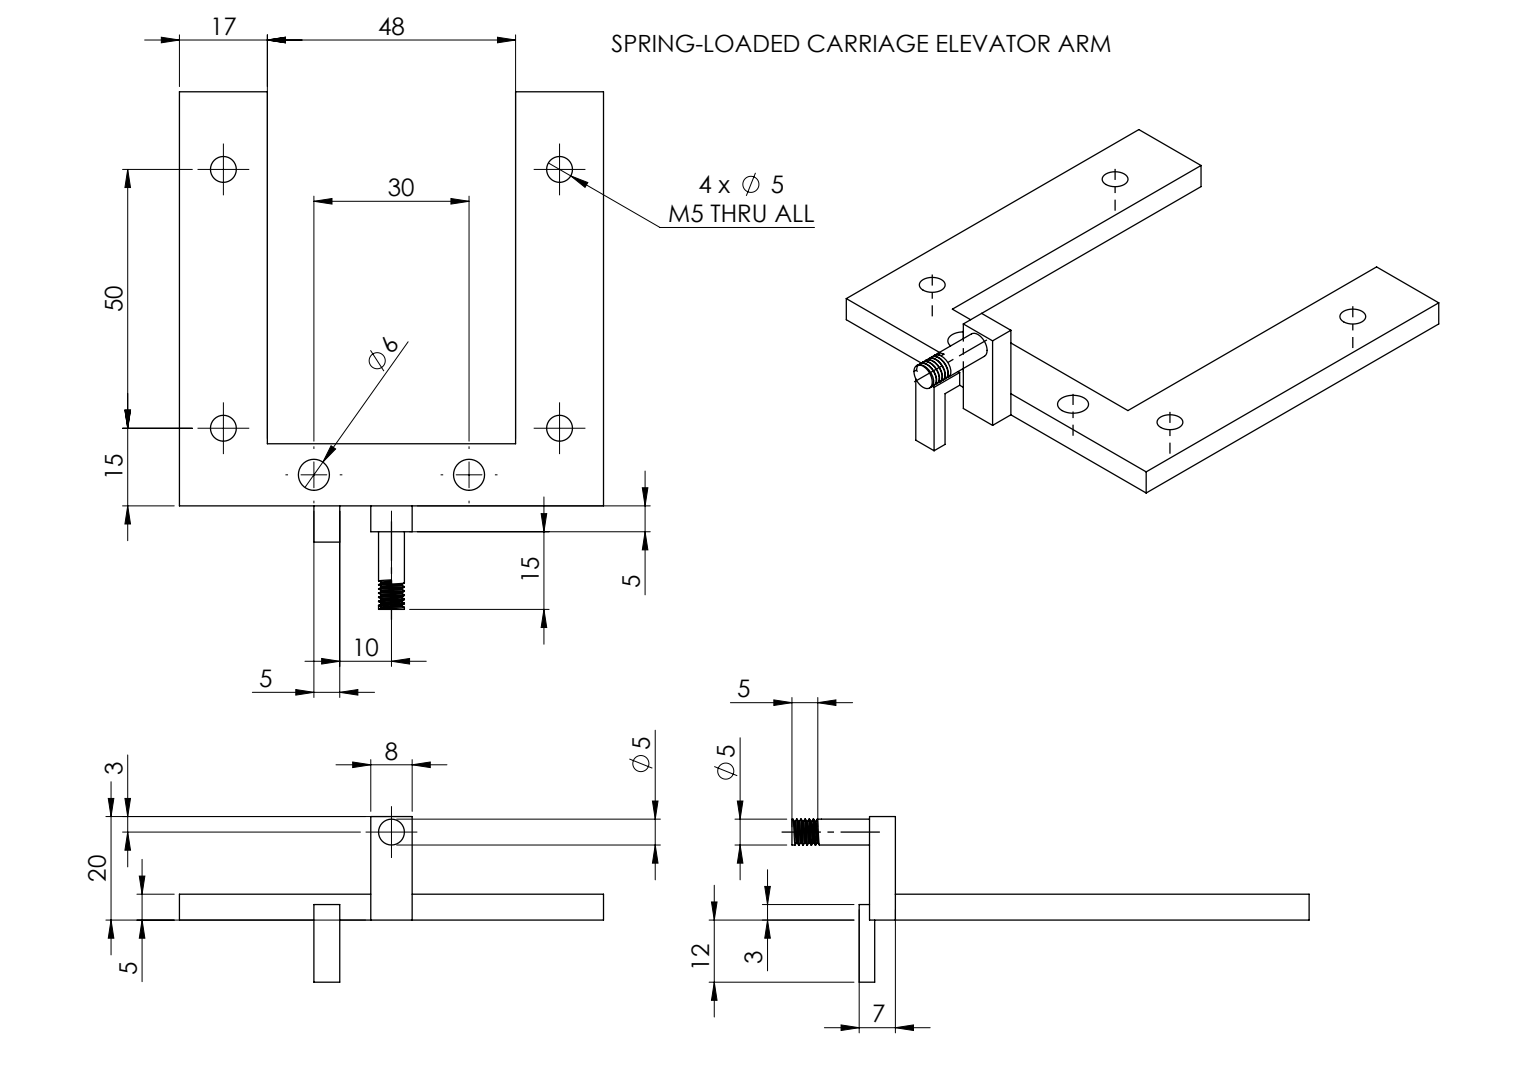
ISO-10303-21;
HEADER;
FILE_DESCRIPTION (('STEP AP214'),
    '1' );
FILE_NAME ('Spring-Loaded Carriage Elevator Arm.step',
    '2026-10-08T14:41:38',
    ( '' ),
    ( '' ),
    'SwSTEP 2.0',
    'SolidWorks 2026',
    '' );
FILE_SCHEMA (( 'AUTOMOTIVE_DESIGN' ));
ENDSEC;

DATA;
#4=DIRECTION ( 'NONE',  ( -0.000000000000000000, 1.000000000000000000, -0.000000000000000000 ) ) ;
#23=DIRECTION ( 'NONE',  ( -0.000000000000000000, -0.000000000000000000, -1.000000000000000000 ) ) ;
#28=CARTESIAN_POINT ( 'NONE',  ( -2.066987300000001415, 63.14382582708705627, 44.80000000109247082 ) ) ;
#31=ORIENTED_EDGE ( 'NONE', *, *, #8748, .T. ) ;
#34=ORIENTED_EDGE ( 'NONE', *, *, #9742, .F. ) ;
#41=CARTESIAN_POINT ( 'NONE',  ( 1.461580736456473684, 65.46158073645646880, 45.45000000109246940 ) ) ;
#50=AXIS2_PLACEMENT_3D ( 'NONE', #5480, #14305, #2436 ) ;
#54=CARTESIAN_POINT ( 'NONE',  ( 1.767766952966369987, 65.76776695296638309, 49.00000000218494023 ) ) ;
#57=EDGE_CURVE ( 'NONE', #1624, #17649, #87, .T. ) ;
#58=CARTESIAN_POINT ( 'NONE',  ( 2.066987300000002303, 63.14382582708705627, 45.30000000109247082 ) ) ;
#68=FACE_OUTER_BOUND ( 'NONE', #2154, .T. ) ;
#73=ORIENTED_EDGE ( 'NONE', *, *, #1505, .T. ) ;
#80=FACE_OUTER_BOUND ( 'NONE', #9007, .T. ) ;
#84=ORIENTED_EDGE ( 'NONE', *, *, #1267, .T. ) ;
#87=LINE ( 'NONE', #2922, #12898 ) ;
#104=CARTESIAN_POINT ( 'NONE',  ( -1.767766952966370209, 65.76776695296638309, 45.09999999999999432 ) ) ;
#108=CARTESIAN_POINT ( 'NONE',  ( 1.035533905932738197, 66.50000000000000000, 47.45000000218494307 ) ) ;
#117=( BOUNDED_SURFACE ( )  B_SPLINE_SURFACE ( 1, 2, ( 
 ( #9163, #1629, #4271, #7495, #8867, #13566, #54, #147, #16622, #6038, #10621, #5837, #11801, #11995, #17795, #6132, #7697, #11700, #4368, #8766, #10328, #18092, #13663, #17993, #16519, #4567, #7300, #3082, #9063, #3189, #15146, #1716, #14852, #17693, #14756, #16325, #2892, #12485, #3479, #12194, #442, #7902, #14057, #8092, #12393, #13866, #14158, #7997, #9347, #18390, #537, #2108, #16718, #6621, #631, #6520, #347, #6427, #4959, #12590, #4862, #4774, #15339, #1815, #3572, #3380, #18195, #18582, #10724, #1916, #2196, #10915, #5055, #16914, #7795, #9453, #10818, #16816, #5148, #11110, #11015, #17106, #3286, #13963, #15243, #15441, #9257, #13766, #15626, #18487, #2006, #6333, #12299, #15537, #18294, #17014, #3670, #9545, #9641, #8190, #6229 ),
 ( #18952, #2384, #1012, #18680, #11198, #18866, #15731, #11580, #14338, #911, #11481, #3953, #5519, #3859, #728, #2668, #5428, #9821, #6987, #17378, #6707, #6893, #8369, #8555, #2573, #12865, #11386, #8648, #2474, #15818, #9915, #14438, #16015, #17201, #1102, #14530, #12953, #14247, #15910, #8462, #7083, #18763, #5245, #17469, #2291, #4045, #17293, #12678, #13046, #3766, #10011, #16101, #19045, #5618, #17578, #8277, #4155, #5336, #11297, #10105, #9735, #818, #6803, #12767, #2961, #4248, #7378, #13151, #17669, #4646, #7471, #2867, #14730, #10206, #4543, #16197, #1401, #10502, #1308, #8739, #4344, #15028, #11876, #7281, #16500, #9040, #13444, #16295, #14933, #19149, #5720, #13349, #2764, #6109, #13247, #28, #19343, #10403, #19244, #1504, #12075 ) ),
 .UNSPECIFIED., .F., .F., .F. ) 
 B_SPLINE_SURFACE_WITH_KNOTS ( ( 2, 2 ),
 ( 3, 2, 2, 2, 2, 2, 2, 2, 2, 2, 2, 2, 2, 2, 2, 2, 2, 2, 2, 2, 2, 2, 2, 2, 2, 2, 2, 2, 2, 2, 2, 2, 2, 2, 2, 2, 2, 2, 2, 2, 2, 2, 2, 2, 2, 2, 2, 2, 2, 2, 3 ),
 ( 0.000000000000000000, 1.000000000000000000 ),
 ( 0.000000000000000000, 0.01785714285714285615, 0.03571428571428571230, 0.05357142857142856845, 0.07142857142857142461, 0.08928571428571428770, 0.1071428571428571369, 0.1250000000000000000, 0.1428571428571428492, 0.1607142857142857262, 0.1785714285714285754, 0.1964285714285714246, 0.2142857142857142738, 0.2321428571428571508, 0.2500000000000000000, 0.2678571428571428492, 0.2857142857142856984, 0.3035714285714285476, 0.3214285714285714524, 0.3392857142857143016, 0.3571428571428571508, 0.3750000000000000000, 0.3928571428571428492, 0.4107142857142856984, 0.4285714285714285476, 0.4464285714285714524, 0.4642857142857143016, 0.4821428571428571508, 0.5000000000000000000, 0.5178571428571429047, 0.5357142857142856984, 0.5535714285714286031, 0.5714285714285713969, 0.5892857142857143016, 0.6071428571428570953, 0.6250000000000000000, 0.6428571428571429047, 0.6607142857142856984, 0.6785714285714286031, 0.6964285714285713969, 0.7142857142857143016, 0.7321428571428570953, 0.7500000000000000000, 0.7678571428571429047, 0.7857142857142856984, 0.8035714285714286031, 0.8214285714285713969, 0.8392857142857143016, 0.8571428571428570953, 0.8750000000000000000, 0.8928571428571429047 ),
 .UNSPECIFIED. ) 
 GEOMETRIC_REPRESENTATION_ITEM ( )  RATIONAL_B_SPLINE_SURFACE ( (
 ( 1.000000000000000000, 0.9238795325112867385, 1.000000000000000000, 0.9238795325112867385, 1.000000000000000000, 0.9238795325112867385, 1.000000000000000000, 0.9238795325112867385, 1.000000000000000000, 0.9238795325112867385, 1.000000000000000000, 0.9238795325112867385, 1.000000000000000000, 0.9238795325112867385, 1.000000000000000000, 0.9238795325112867385, 1.000000000000000000, 0.9238795325112867385, 1.000000000000000000, 0.9238795325112867385, 1.000000000000000000, 0.9238795325112867385, 1.000000000000000000, 0.9238795325112867385, 1.000000000000000000, 0.9238795325112867385, 1.000000000000000000, 0.9238795325112867385, 1.000000000000000000, 0.9238795325112867385, 1.000000000000000000, 0.9238795325112867385, 1.000000000000000000, 0.9238795325112867385, 1.000000000000000000, 0.9238795325112867385, 1.000000000000000000, 0.9238795325112867385, 1.000000000000000000, 0.9238795325112867385, 1.000000000000000000, 0.9238795325112867385, 1.000000000000000000, 0.9238795325112867385, 1.000000000000000000, 0.9238795325112867385, 1.000000000000000000, 0.9238795325112867385, 1.000000000000000000, 0.9238795325112867385, 1.000000000000000000, 0.9238795325112867385, 1.000000000000000000, 0.9238795325112867385, 1.000000000000000000, 0.9238795325112867385, 1.000000000000000000, 0.9238795325112867385, 1.000000000000000000, 0.9238795325112867385, 1.000000000000000000, 0.9238795325112867385, 1.000000000000000000, 0.9238795325112867385, 1.000000000000000000, 0.9238795325112867385, 1.000000000000000000, 0.9238795325112867385, 1.000000000000000000, 0.9238795325112867385, 1.000000000000000000, 0.9238795325112867385, 1.000000000000000000, 0.9238795325112867385, 1.000000000000000000, 0.9238795325112867385, 1.000000000000000000, 0.9238795325112867385, 1.000000000000000000, 0.9238795325112867385, 1.000000000000000000, 0.9238795325112867385, 1.000000000000000000, 0.9238795325112867385, 1.000000000000000000, 0.9238795325112867385, 1.000000000000000000, 0.9238795325112867385, 1.000000000000000000, 0.9238795325112867385, 1.000000000000000000, 0.9238795325112867385, 1.000000000000000000, 0.9238795325112867385, 1.000000000000000000, 0.9238795325112867385, 1.000000000000000000, 0.9238795325112867385, 1.000000000000000000, 0.9238795325112867385, 1.000000000000000000),
 ( 1.000000000000000000, 0.9238795325112867385, 1.000000000000000000, 0.9238795325112867385, 1.000000000000000000, 0.9238795325112867385, 1.000000000000000000, 0.9238795325112867385, 1.000000000000000000, 0.9238795325112867385, 1.000000000000000000, 0.9238795325112867385, 1.000000000000000000, 0.9238795325112867385, 1.000000000000000000, 0.9238795325112867385, 1.000000000000000000, 0.9238795325112867385, 1.000000000000000000, 0.9238795325112867385, 1.000000000000000000, 0.9238795325112867385, 1.000000000000000000, 0.9238795325112867385, 1.000000000000000000, 0.9238795325112867385, 1.000000000000000000, 0.9238795325112867385, 1.000000000000000000, 0.9238795325112867385, 1.000000000000000000, 0.9238795325112867385, 1.000000000000000000, 0.9238795325112867385, 1.000000000000000000, 0.9238795325112867385, 1.000000000000000000, 0.9238795325112867385, 1.000000000000000000, 0.9238795325112867385, 1.000000000000000000, 0.9238795325112867385, 1.000000000000000000, 0.9238795325112867385, 1.000000000000000000, 0.9238795325112867385, 1.000000000000000000, 0.9238795325112867385, 1.000000000000000000, 0.9238795325112867385, 1.000000000000000000, 0.9238795325112867385, 1.000000000000000000, 0.9238795325112867385, 1.000000000000000000, 0.9238795325112867385, 1.000000000000000000, 0.9238795325112867385, 1.000000000000000000, 0.9238795325112867385, 1.000000000000000000, 0.9238795325112867385, 1.000000000000000000, 0.9238795325112867385, 1.000000000000000000, 0.9238795325112867385, 1.000000000000000000, 0.9238795325112867385, 1.000000000000000000, 0.9238795325112867385, 1.000000000000000000, 0.9238795325112867385, 1.000000000000000000, 0.9238795325112867385, 1.000000000000000000, 0.9238795325112867385, 1.000000000000000000, 0.9238795325112867385, 1.000000000000000000, 0.9238795325112867385, 1.000000000000000000, 0.9238795325112867385, 1.000000000000000000, 0.9238795325112867385, 1.000000000000000000, 0.9238795325112867385, 1.000000000000000000, 0.9238795325112867385, 1.000000000000000000, 0.9238795325112867385, 1.000000000000000000, 0.9238795325112867385, 1.000000000000000000, 0.9238795325112867385, 1.000000000000000000, 0.9238795325112867385, 1.000000000000000000, 0.9238795325112867385, 1.000000000000000000, 0.9238795325112867385, 1.000000000000000000) ) ) 
 REPRESENTATION_ITEM ( '' )  SURFACE ( )  );
#121=DIRECTION ( 'NONE',  ( -0.000000000000000000, -1.000000000000000000, -0.000000000000000000 ) ) ;
#127=DIRECTION ( 'NONE',  ( -0.000000000000000000, -0.000000000000000000, -1.000000000000000000 ) ) ;
#131=DIRECTION ( 'NONE',  ( -0.000000000000000000, -0.000000000000000000, -1.000000000000000000 ) ) ;
#137=CARTESIAN_POINT ( 'NONE',  ( -2.066987300000001415, 64.85617417291294373, 48.10000000109246798 ) ) ;
#142=ORIENTED_EDGE ( 'NONE', *, *, #12510, .F. ) ;
#147=CARTESIAN_POINT ( 'NONE',  ( 2.500000000000001776, 65.03553390593273775, 48.95000000218495018 ) ) ;
#156=CARTESIAN_POINT ( 'NONE',  ( -2.066987300000001859, 64.85617417291294373, 48.90000000109247225 ) ) ;
#159=PLANE ( 'NONE',  #4117 ) ;
#165=EDGE_CURVE ( 'NONE', #16279, #13992, #8531, .T. ) ;
#186=CARTESIAN_POINT ( 'NONE',  ( 0.000000000000000000, 47.00000000000000711, -50.00000000000000000 ) ) ;
#195=ORIENTED_EDGE ( 'NONE', *, *, #2336, .T. ) ;
#203=CARTESIAN_POINT ( 'NONE',  ( 0.8561741729129471734, 61.93301270000000613, 49.00000000109246656 ) ) ;
#204=DIRECTION ( 'NONE',  ( 0.000000000000000000, 0.000000000000000000, 1.000000000000000000 ) ) ;
#208=CARTESIAN_POINT ( 'NONE',  ( -2.500000000000001776, 64.00000000000000000, 44.50000000218494733 ) ) ;
#211=LINE ( 'NONE', #15300, #5330 ) ;
#213=CARTESIAN_POINT ( 'NONE',  ( -2.500000000000001776, 64.00000000000000000, 46.79999999999999716 ) ) ;
#215=CARTESIAN_POINT ( 'NONE',  ( -10.00000000000000000, 50.00000000000000000, 30.00000000000000000 ) ) ;
#220=CARTESIAN_POINT ( 'NONE',  ( -2.500000000000019096, 65.03553390593272354, 48.35000000000000853 ) ) ;
#225=AXIS2_PLACEMENT_3D ( 'NONE', #6440, #18405, #16930 ) ;
#227=DIRECTION ( 'NONE',  ( 0.000000000000000000, 0.000000000000000000, -1.000000000000000000 ) ) ;
#232=VERTEX_POINT ( 'NONE', #15660 ) ;
#240=CARTESIAN_POINT ( 'NONE',  ( -32.50000000000000000, 52.00000000000000711, 12.50000000000000000 ) ) ;
#251=DIRECTION ( 'NONE',  ( -0.000000000000000000, -0.000000000000000000, -1.000000000000000000 ) ) ;
#253=CARTESIAN_POINT ( 'NONE',  ( 2.066987300000001859, 64.85617417291294373, 46.20000000109247651 ) ) ;
#261=ORIENTED_EDGE ( 'NONE', *, *, #4730, .T. ) ;
#272=ORIENTED_EDGE ( 'NONE', *, *, #12825, .F. ) ;
#274=DIRECTION ( 'NONE',  ( -1.000000000000000000, 0.000000000000000000, 0.000000000000000000 ) ) ;
#292=VERTEX_POINT ( 'NONE', #6652 ) ;
#295=CARTESIAN_POINT ( 'NONE',  ( 2.066987300000001415, 64.85617417291294373, 49.20000000109247651 ) ) ;
#297=VERTEX_POINT ( 'NONE', #14188 ) ;
#307=LINE ( 'NONE', #9221, #11899 ) ;
#311=DIRECTION ( 'NONE',  ( 1.000000000000000000, 0.000000000000000000, 0.000000000000000000 ) ) ;
#318=AXIS2_PLACEMENT_3D ( 'NONE', #6383, #18632, #12346 ) ;
#323=CARTESIAN_POINT ( 'NONE',  ( -10.00000000000000000, 0.000000000000000000, 33.99999999999999289 ) ) ;
#324=ORIENTED_EDGE ( 'NONE', *, *, #4947, .F. ) ;
#333=ORIENTED_EDGE ( 'NONE', *, *, #12310, .F. ) ;
#341=DIRECTION ( 'NONE',  ( -0.000000000000000000, -1.000000000000000000, 0.000000000000000000 ) ) ;
#347=CARTESIAN_POINT ( 'NONE',  ( 2.500000000000001776, 64.00000000000000000, 46.50000000218494733 ) ) ;
#354=FACE_OUTER_BOUND ( 'NONE', #14089, .T. ) ;
#355=( GEOMETRIC_REPRESENTATION_CONTEXT ( 3 ) GLOBAL_UNCERTAINTY_ASSIGNED_CONTEXT ( ( #18086 ) ) GLOBAL_UNIT_ASSIGNED_CONTEXT ( ( #12843, #5500, #19029 ) ) REPRESENTATION_CONTEXT ( 'NONE', 'WORKASPACE' ) );
#356=CARTESIAN_POINT ( 'NONE',  ( -2.066987300000001415, 63.14382582708705627, 48.20000000109247651 ) ) ;
#362=AXIS2_PLACEMENT_3D ( 'NONE', #17371, #11102, #3758 ) ;
#375=VERTEX_POINT ( 'NONE', #7113 ) ;
#387=EDGE_CURVE ( 'NONE', #7750, #14031, #2123, .T. ) ;
#395=EDGE_LOOP ( 'NONE', ( #10179, #10468 ) ) ;
#399=CARTESIAN_POINT ( 'NONE',  ( -0.8561741729129466183, 61.93301270000000613, 47.30000000109247082 ) ) ;
#400=FACE_OUTER_BOUND ( 'NONE', #585, .T. ) ;
#406=ORIENTED_EDGE ( 'NONE', *, *, #3062, .T. ) ;
#419=ORIENTED_EDGE ( 'NONE', *, *, #16592, .T. ) ;
#420=EDGE_CURVE ( 'NONE', #9430, #8882, #10133, .T. ) ;
#434=DIRECTION ( 'NONE',  ( -0.000000000000000000, 1.000000000000000000, -0.000000000000000000 ) ) ;
#439=UNCERTAINTY_MEASURE_WITH_UNIT (LENGTH_MEASURE( 1.000000000000000082E-05 ), #14477, 'distance_accuracy_value', 'NONE');
#442=CARTESIAN_POINT ( 'NONE',  ( 2.500000000000001776, 64.00000000000000000, 47.30000000218494449 ) ) ;
#444=DIRECTION ( 'NONE',  ( -0.000000000000000000, -0.000000000000000000, -1.000000000000000000 ) ) ;
#450=CARTESIAN_POINT ( 'NONE',  ( 1.461580736456473684, 65.46158073645646880, 48.65000000109247225 ) ) ;
#454=CYLINDRICAL_SURFACE ( 'NONE', #225, 2.999999999999999112 ) ;
#457=VECTOR ( 'NONE', #7788, 1000.000000000000000 ) ;
#459=ORIENTED_EDGE ( 'NONE', *, *, #7687, .F. ) ;
#466=CARTESIAN_POINT ( 'NONE',  ( 1.461580736456473684, 65.46158073645646880, 45.25000000109247367 ) ) ;
#490=CARTESIAN_POINT ( 'NONE',  ( -2.066987300000001415, 64.00000000000000000, 49.55000000109247082 ) ) ;
#498=DIRECTION ( 'NONE',  ( 1.000000000000000000, 0.000000000000000000, -0.000000000000000000 ) ) ;
#505=CARTESIAN_POINT ( 'NONE',  ( -1.767766952966370209, 65.76776695296638309, 49.20000000218494307 ) ) ;
#537=CARTESIAN_POINT ( 'NONE',  ( -1.767766952966370209, 65.76776695296638309, 46.80000000218494449 ) ) ;
#543=DIRECTION ( 'NONE',  ( 0.000000000000000000, 0.000000000000000000, 1.000000000000000000 ) ) ;
#546=CARTESIAN_POINT ( 'NONE',  ( 1.461580736456473684, 65.46158073645646880, 47.85000000109246798 ) ) ;
#552=ORIENTED_EDGE ( 'NONE', *, *, #4349, .F. ) ;
#560=CARTESIAN_POINT ( 'NONE',  ( 2.066987300000002303, 63.14382582708705627, 47.50000000109246656 ) ) ;
#583=CARTESIAN_POINT ( 'NONE',  ( 0.8561741729129460632, 66.06698730000000808, 49.30000000109246372 ) ) ;
#585=EDGE_LOOP ( 'NONE', ( #18934, #14409, #5001, #12417 ) ) ;
#611=ORIENTED_EDGE ( 'NONE', *, *, #18614, .F. ) ;
#618=CARTESIAN_POINT ( 'NONE',  ( 1.767766952966370653, 62.23223304703363112, 46.29999999999999716 ) ) ;
#624=DIRECTION ( 'NONE',  ( -0.000000000000000000, 1.000000000000000000, -0.000000000000000000 ) ) ;
#631=CARTESIAN_POINT ( 'NONE',  ( 1.767766952966369987, 65.76776695296638309, 46.60000000218494165 ) ) ;
#642=CARTESIAN_POINT ( 'NONE',  ( -2.066987300000001859, 64.85617417291294373, 45.70000000109248361 ) ) ;
#646=LINE ( 'NONE', #13977, #4274 ) ;
#652=CIRCLE ( 'NONE', #5974, 2.999999999999999112 ) ;
#662=CARTESIAN_POINT ( 'NONE',  ( 0.8561741729129460632, 66.06698729999999387, 46.90000000109247225 ) ) ;
#698=CARTESIAN_POINT ( 'NONE',  ( 0.000000000000000000, 0.000000000000000000, -50.00000000000000000 ) ) ;
#715=ORIENTED_EDGE ( 'NONE', *, *, #16980, .F. ) ;
#719=CARTESIAN_POINT ( 'NONE',  ( -1.035533905932738863, 61.50000000000000000, 46.14999999999999858 ) ) ;
#720=CARTESIAN_POINT ( 'NONE',  ( -2.500000000000001776, 64.00000000000000000, 46.10000000218494165 ) ) ;
#728=CARTESIAN_POINT ( 'NONE',  ( -1.461580736456473462, 62.53841926354353120, 48.85000000109246798 ) ) ;
#730=DIRECTION ( 'NONE',  ( -1.000000000000000000, 0.000000000000000000, 0.000000000000000000 ) ) ;
#732=ADVANCED_FACE ( 'NONE', ( #1925 ), #15252, .T. ) ;
#737=CARTESIAN_POINT ( 'NONE',  ( 1.461580736456473684, 65.46158073645646880, 45.45000000109246940 ) ) ;
#745=CARTESIAN_POINT ( 'NONE',  ( -1.461580736456473462, 62.53841926354353120, 46.45000000109246940 ) ) ;
#749=CARTESIAN_POINT ( 'NONE',  ( 2.066987300000002303, 63.14382582708705627, 45.90000000109247225 ) ) ;
#756=EDGE_CURVE ( 'NONE', #8924, #4687, #13097, .T. ) ;
#771=CARTESIAN_POINT ( 'NONE',  ( 1.035533905932738197, 66.50000000000000000, 47.34999999999998721 ) ) ;
#782=DIRECTION ( 'NONE',  ( -0.000000000000000000, -0.000000000000000000, -1.000000000000000000 ) ) ;
#787=DIRECTION ( 'NONE',  ( 0.000000000000000000, 1.000000000000000000, 0.000000000000000000 ) ) ;
#792=ORIENTED_EDGE ( 'NONE', *, *, #7610, .F. ) ;
#808=DIRECTION ( 'NONE',  ( -0.000000000000000000, -0.000000000000000000, -1.000000000000000000 ) ) ;
#818=CARTESIAN_POINT ( 'NONE',  ( -0.8561741729129465073, 61.93301270000000613, 46.50000000109247367 ) ) ;
#829=CARTESIAN_POINT ( 'NONE',  ( -1.767766952966370209, 65.76776695296638309, 48.29999999999999716 ) ) ;
#837=CARTESIAN_POINT ( 'NONE',  ( 1.461580736456473906, 62.53841926354353120, 46.65000000109247225 ) ) ;
#841=CARTESIAN_POINT ( 'NONE',  ( -1.461580736456473906, 65.46158073645646880, 47.05000000109247082 ) ) ;
#849=CARTESIAN_POINT ( 'NONE',  ( 2.500000000000001776, 64.00000000000000000, 47.99999999999999289 ) ) ;
#851=EDGE_CURVE ( 'NONE', #13992, #16279, #14676, .T. ) ;
#902=DIRECTION ( 'NONE',  ( -0.000000000000000000, -1.000000000000000000, -0.000000000000000000 ) ) ;
#905=CARTESIAN_POINT ( 'NONE',  ( -15.00000000000000000, 50.00000000000000000, 30.00000000000000000 ) ) ;
#908=VERTEX_POINT ( 'NONE', #18961 ) ;
#911=CARTESIAN_POINT ( 'NONE',  ( 2.066987300000002303, 63.14382582708705627, 49.10000000109246088 ) ) ;
#917=AXIS2_PLACEMENT_3D ( 'NONE', #6913, #14180, #12886 ) ;
#921=CARTESIAN_POINT ( 'NONE',  ( -0.8561741729129465073, 61.93301270000000613, 45.10000000109246798 ) ) ;
#922=DIRECTION ( 'NONE',  ( 0.000000000000000000, 1.000000000000000000, 0.000000000000000000 ) ) ;
#925=CARTESIAN_POINT ( 'NONE',  ( -2.500000000000001776, 64.00000000000000000, 48.50000000218494023 ) ) ;
#929=EDGE_LOOP ( 'NONE', ( #4729, #17644, #6889, #19102, #1362, #1856, #1672, #7418 ) ) ;
#931=CARTESIAN_POINT ( 'NONE',  ( -2.066987300000001415, 64.00000000000000000, 45.55000000109246372 ) ) ;
#932=AXIS2_PLACEMENT_3D ( 'NONE', #16950, #3411, #7830 ) ;
#937=CARTESIAN_POINT ( 'NONE',  ( 1.461580736456473906, 62.53841926354353120, 49.25000000109246656 ) ) ;
#946=DIRECTION ( 'NONE',  ( 0.000000000000000000, -1.000000000000000000, 0.000000000000000000 ) ) ;
#955=ORIENTED_EDGE ( 'NONE', *, *, #6127, .F. ) ;
#958=EDGE_CURVE ( 'NONE', #6376, #15290, #14540, .T. ) ;
#964=VERTEX_POINT ( 'NONE', #8284 ) ;
#966=( BOUNDED_CURVE ( )  B_SPLINE_CURVE ( 2, ( #11278, #18750, #6971, #15996, #1084, #12938, #18933, #13032, #5598 ),
 .UNSPECIFIED., .F., .F. ) 
 B_SPLINE_CURVE_WITH_KNOTS ( ( 3, 2, 2, 2, 3 ),
 ( 0.4285714285714284366, 0.4464285714285713413, 0.4642857142857141906, 0.4821428571428570953, 0.4999999999999999445 ),
 .UNSPECIFIED. ) 
 CURVE ( )  GEOMETRIC_REPRESENTATION_ITEM ( )  RATIONAL_B_SPLINE_CURVE ( ( 1.000000000000000444, 0.9238795325112862944, 1.000000000000000000, 0.9238795325112867385, 1.000000000000000000, 0.9238795325112867385, 1.000000000000000000, 0.9238795325112869605, 0.9999999999999997780 ) ) 
 REPRESENTATION_ITEM ( '' )  );
#969=ORIENTED_EDGE ( 'NONE', *, *, #5225, .T. ) ;
#979=VECTOR ( 'NONE', #4332, 1000.000000000000000 ) ;
#999=AXIS2_PLACEMENT_3D ( 'NONE', #7203, #19169, #14462 ) ;
#1000=CARTESIAN_POINT ( 'NONE',  ( 3.999999999999998224, 67.00000000000000000, 34.99999999999999289 ) ) ;
#1001=EDGE_CURVE ( 'NONE', #15589, #6260, #11589, .T. ) ;
#1012=CARTESIAN_POINT ( 'NONE',  ( -1.461580736456473906, 65.46158073645646880, 49.45000000109246940 ) ) ;
#1016=CLOSED_SHELL ( 'NONE', ( #2998, #16570, #3537, #10721, #5242, #6217, #13298, #18724, #17316, #1952, #11913, #18660, #732, #7313, #10539, #10222, #3338, #15764, #15018, #3137, #11666, #4956, #6976, #2789, #8547, #1023, #10419, #4151, #13881, #18461, #11109, #4449, #9828, #10820, #2175, #10845, #14410, #10785, #8215, #11618, #5050, #3662, #4463, #9985, #5280, #5699, #11404, #10916, #6266, #18784, #14503, #7001, #3782, #14357 ) ) ;
#1020=CARTESIAN_POINT ( 'NONE',  ( -2.500000000000006661, 65.03553390593272354, 45.25000000218494733 ) ) ;
#1023=ADVANCED_FACE ( 'NONE', ( #7290, #12355, #16508, #9050, #16406, #10215, #5823 ), #19158, .T. ) ;
#1025=CARTESIAN_POINT ( 'NONE',  ( 4.592425496802577917E-16, 61.50000000000000000, 48.59999999999999432 ) ) ;
#1032=CARTESIAN_POINT ( 'NONE',  ( 2.066987300000001415, 64.00000000000000000, 45.15000000109247225 ) ) ;
#1036=CARTESIAN_POINT ( 'NONE',  ( 2.066987300000002303, 63.14382582708705627, 48.50000000109246656 ) ) ;
#1038=CARTESIAN_POINT ( 'NONE',  ( -2.500000000000001776, 64.00000000000000000, 45.30000000218493739 ) ) ;
#1044=CARTESIAN_POINT ( 'NONE',  ( 2.500000000000002220, 62.96446609406726225, 44.85000000218494165 ) ) ;
#1048=FILL_AREA_STYLE ('',( #3808 ) ) ;
#1065=LINE ( 'NONE', #19012, #11851 ) ;
#1079=CARTESIAN_POINT ( 'NONE',  ( -1.035533905932738863, 61.50000000000000000, 45.34999999999999432 ) ) ;
#1080=ORIENTED_EDGE ( 'NONE', *, *, #9742, .T. ) ;
#1082=CARTESIAN_POINT ( 'NONE',  ( -1.530808498934192803E-16, 66.50000000000000000, 48.99999999999999289 ) ) ;
#1084=CARTESIAN_POINT ( 'NONE',  ( -1.530808498934192803E-16, 66.50000000000000000, 46.70000000218494307 ) ) ;
#1089=CARTESIAN_POINT ( 'NONE',  ( -2.500000000000001776, 64.00000000000000000, 47.70000000218494307 ) ) ;
#1090=CIRCLE ( 'NONE', #16120, 2.999999999999999112 ) ;
#1091=CARTESIAN_POINT ( 'NONE',  ( -1.767766952966370209, 65.76776695296638309, 48.40000000218494591 ) ) ;
#1102=CARTESIAN_POINT ( 'NONE',  ( -1.461580736456473906, 65.46158073645646880, 47.85000000109246798 ) ) ;
#1107=CARTESIAN_POINT ( 'NONE',  ( -1.767766952966369765, 62.23223304703363112, 46.20000000218494307 ) ) ;
#1113=CARTESIAN_POINT ( 'NONE',  ( -2.500000000000001776, 64.00000000000000000, 49.99999999999999289 ) ) ;
#1115=CARTESIAN_POINT ( 'NONE',  ( 1.767766952966369987, 65.76776695296638309, 46.49999999999999289 ) ) ;
#1116=CARTESIAN_POINT ( 'NONE',  ( -2.066987300000001415, 64.85617417291294373, 49.70000000109247651 ) ) ;
#1118=VECTOR ( 'NONE', #7896, 1000.000000000000000 ) ;
#1126=DIRECTION ( 'NONE',  ( -2.602085213965211135E-16, 1.000000000000000000, 0.000000000000000000 ) ) ;
#1131=CARTESIAN_POINT ( 'NONE',  ( 1.461580736456473906, 62.53841926354353120, 47.65000000109247225 ) ) ;
#1148=ORIENTED_EDGE ( 'NONE', *, *, #17670, .T. ) ;
#1149=ORIENTED_EDGE ( 'NONE', *, *, #13711, .F. ) ;
#1178=CARTESIAN_POINT ( 'NONE',  ( -2.499999999999999112, 65.03553390593273775, 49.15000000000000568 ) ) ;
#1181=EDGE_LOOP ( 'NONE', ( #272, #18537, #17775, #4023 ) ) ;
#1186=DIRECTION ( 'NONE',  ( 1.000000000000000000, 0.000000000000000000, 0.000000000000000000 ) ) ;
#1190=CARTESIAN_POINT ( 'NONE',  ( 0.000000000000000000, 0.000000000000000000, 18.00000000000000000 ) ) ;
#1198=VECTOR ( 'NONE', #922, 1000.000000000000000 ) ;
#1202=DIRECTION ( 'NONE',  ( -0.000000000000000000, -1.000000000000000000, -0.000000000000000000 ) ) ;
#1208=CARTESIAN_POINT ( 'NONE',  ( 1.767766952966370653, 62.23223304703363112, 46.29999999999999716 ) ) ;
#1209=CARTESIAN_POINT ( 'NONE',  ( 2.066987300000001859, 63.14382582708704916, 48.50000000109246656 ) ) ;
#1216=EDGE_LOOP ( 'NONE', ( #11012, #8822 ) ) ;
#1224=CARTESIAN_POINT ( 'NONE',  ( -0.8561741729129465073, 61.93301270000000613, 49.10000000109246088 ) ) ;
#1252=( BOUNDED_CURVE ( )  B_SPLINE_CURVE ( 2, ( #7047, #18828, #13216, #13113, #2628, #11737, #14599, #7248, #5401 ),
 .UNSPECIFIED., .F., .F. ) 
 B_SPLINE_CURVE_WITH_KNOTS ( ( 3, 2, 2, 2, 3 ),
 ( 0.3571428571428571508, 0.3750000000000000000, 0.3928571428571427937, 0.4107142857142855874, 0.4285714285714284366 ),
 .UNSPECIFIED. ) 
 CURVE ( )  GEOMETRIC_REPRESENTATION_ITEM ( )  RATIONAL_B_SPLINE_CURVE ( ( 1.000000000000000000, 0.9238795325112867385, 1.000000000000000000, 0.9238795325112867385, 1.000000000000000000, 0.9238795325112867385, 1.000000000000000000, 0.9238795325112871826, 0.9999999999999995559 ) ) 
 REPRESENTATION_ITEM ( '' )  );
#1261=ORIENTED_EDGE ( 'NONE', *, *, #15118, .T. ) ;
#1264=DIRECTION ( 'NONE',  ( -0.000000000000000000, -0.000000000000000000, -1.000000000000000000 ) ) ;
#1267=EDGE_CURVE ( 'NONE', #964, #16382, #6768, .T. ) ;
#1271=CARTESIAN_POINT ( 'NONE',  ( -41.00000000000000000, 47.00000000000000711, 30.00000000000000000 ) ) ;
#1285=CARTESIAN_POINT ( 'NONE',  ( -2.499999999999992450, 65.03553390593275196, 47.65000000218494591 ) ) ;
#1293=CARTESIAN_POINT ( 'NONE',  ( -1.530808498934192803E-16, 66.50000000000000000, 44.30000000218494449 ) ) ;
#1308=CARTESIAN_POINT ( 'NONE',  ( -1.461580736456473462, 62.53841926354353120, 45.65000000109247225 ) ) ;
#1313=DIRECTION ( 'NONE',  ( -1.000000000000000000, 0.000000000000000000, 0.000000000000000000 ) ) ;
#1320=CARTESIAN_POINT ( 'NONE',  ( -1.767766952966369765, 62.23223304703363112, 47.69999999999999574 ) ) ;
#1321=CARTESIAN_POINT ( 'NONE',  ( 0.8561741729129471734, 61.93301270000000613, 47.60000000109246798 ) ) ;
#1326=ORIENTED_EDGE ( 'NONE', *, *, #6127, .T. ) ;
#1332=CARTESIAN_POINT ( 'NONE',  ( 2.066987300000001859, 64.85617417291294373, 46.20000000109247651 ) ) ;
#1341=LINE ( 'NONE', #7511, #15382 ) ;
#1348=FACE_OUTER_BOUND ( 'NONE', #929, .T. ) ;
#1354=CARTESIAN_POINT ( 'NONE',  ( -2.500000000000001776, 64.00000000000000000, 49.99999999999999289 ) ) ;
#1358=CARTESIAN_POINT ( 'NONE',  ( 1.035533905932739751, 61.50000000000000000, 47.04999999999999716 ) ) ;
#1362=ORIENTED_EDGE ( 'NONE', *, *, #9857, .T. ) ;
#1363=CARTESIAN_POINT ( 'NONE',  ( 1.035533905932738197, 66.50000000000000000, 45.75000000000000000 ) ) ;
#1383=EDGE_LOOP ( 'NONE', ( #16169, #261 ) ) ;
#1401=CARTESIAN_POINT ( 'NONE',  ( 3.796994071234847710E-16, 61.93301269999999903, 45.75000000109247367 ) ) ;
#1411=DIRECTION ( 'NONE',  ( 0.000000000000000000, 0.000000000000000000, 1.000000000000000000 ) ) ;
#1414=CARTESIAN_POINT ( 'NONE',  ( 2.500000000000002220, 62.96446609406726935, 46.34999999999999432 ) ) ;
#1415=CARTESIAN_POINT ( 'NONE',  ( 0.8561741729129460632, 66.06698730000000808, 47.90000000109247225 ) ) ;
#1427=CARTESIAN_POINT ( 'NONE',  ( -1.265664690411616068E-16, 66.06698730000000808, 46.35000000109246798 ) ) ;
#1435=DIRECTION ( 'NONE',  ( -0.000000000000000000, 0.000000000000000000, 1.000000000000000000 ) ) ;
#1451=FACE_OUTER_BOUND ( 'NONE', #7733, .T. ) ;
#1453=CARTESIAN_POINT ( 'NONE',  ( 2.066987300000001859, 64.85617417291294373, 48.40000000109247225 ) ) ;
#1455=ORIENTED_EDGE ( 'NONE', *, *, #8671, .T. ) ;
#1456=ORIENTED_EDGE ( 'NONE', *, *, #16499, .T. ) ;
#1495=( BOUNDED_CURVE ( )  B_SPLINE_CURVE ( 2, ( #13526, #5696, #104, #7154, #11657 ),
 .UNSPECIFIED., .F., .F. ) 
 B_SPLINE_CURVE_WITH_KNOTS ( ( 3, 2, 3 ),
 ( 0.8571428571428569843, 0.8750000000000000000, 0.8928571428571429047 ),
 .UNSPECIFIED. ) 
 CURVE ( )  GEOMETRIC_REPRESENTATION_ITEM ( )  RATIONAL_B_SPLINE_CURVE ( ( 1.000000000000000444, 0.9238795325112862944, 1.000000000000000000, 0.9238795325112867385, 1.000000000000000000 ) ) 
 REPRESENTATION_ITEM ( '' )  );
#1499=CARTESIAN_POINT ( 'NONE',  ( 0.000000000000000000, 64.00000000000000000, 49.99999999999999289 ) ) ;
#1504=CARTESIAN_POINT ( 'NONE',  ( -0.8561741729129461742, 66.06698729999999387, 44.60000000109246088 ) ) ;
#1505=EDGE_CURVE ( 'NONE', #6482, #5462, #13443, .T. ) ;
#1511=DIRECTION ( 'NONE',  ( -1.000000000000000000, 0.000000000000000000, 0.000000000000000000 ) ) ;
#1516=CARTESIAN_POINT ( 'NONE',  ( 0.8561741729129460632, 66.06698730000000808, 45.50000000109247367 ) ) ;
#1517=ADVANCED_BREP_SHAPE_REPRESENTATION ( '', ( #3741, #1791 ), #13038 ) ;
#1528=CARTESIAN_POINT ( 'NONE',  ( -1.461580736456473906, 65.46158073645646880, 45.65000000109247225 ) ) ;
#1533=CARTESIAN_POINT ( 'NONE',  ( -2.066987300000001859, 64.85617417291294373, 49.70000000109248361 ) ) ;
#1546=ORIENTED_EDGE ( 'NONE', *, *, #14757, .F. ) ;
#1558=CARTESIAN_POINT ( 'NONE',  ( 24.00000000000000000, 52.00000000000000711, -50.00000000000000000 ) ) ;
#1573=AXIS2_PLACEMENT_3D ( 'NONE', #8509, #17622, #14485 ) ;
#1576=EDGE_CURVE ( 'NONE', #19196, #7027, #4207, .T. ) ;
#1583=DIRECTION ( 'NONE',  ( 0.000000000000000000, 0.000000000000000000, 1.000000000000000000 ) ) ;
#1584=EDGE_LOOP ( 'NONE', ( #18929, #14603 ) ) ;
#1587=LINE ( 'NONE', #4230, #13468 ) ;
#1599=DIRECTION ( 'NONE',  ( -1.000000000000000000, 0.000000000000000000, 0.000000000000000000 ) ) ;
#1606=FACE_OUTER_BOUND ( 'NONE', #17122, .T. ) ;
#1609=FACE_OUTER_BOUND ( 'NONE', #7228, .T. ) ;
#1617=EDGE_CURVE ( 'NONE', #14815, #6260, #14889, .T. ) ;
#1618=CARTESIAN_POINT ( 'NONE',  ( 1.461580736456473906, 62.53841926354353120, 46.85000000109246798 ) ) ;
#1622=CARTESIAN_POINT ( 'NONE',  ( -15.00000000000000000, 50.00000000000000711, 37.00000000000000000 ) ) ;
#1624=VERTEX_POINT ( 'NONE', #4506 ) ;
#1629=CARTESIAN_POINT ( 'NONE',  ( -2.500000000000001776, 65.03553390593273775, 49.25000000218494023 ) ) ;
#1638=CARTESIAN_POINT ( 'NONE',  ( 0.8561741729129460632, 66.06698729999999387, 47.90000000109247225 ) ) ;
#1649=PLANE ( 'NONE',  #18504 ) ;
#1655=CARTESIAN_POINT ( 'NONE',  ( 0.8561741729129460632, 66.06698729999999387, 48.50000000109246656 ) ) ;
#1663=DIRECTION ( 'NONE',  ( -1.000000000000000000, -6.123233995736588542E-17, 0.000000000000000000 ) ) ;
#1672=ORIENTED_EDGE ( 'NONE', *, *, #15752, .T. ) ;
#1675=CARTESIAN_POINT ( 'NONE',  ( 2.066987300000001415, 64.85617417291294373, 48.40000000109247225 ) ) ;
#1691=CARTESIAN_POINT ( 'NONE',  ( 14.99999999999998579, 47.00000000000000711, 23.99999999999997158 ) ) ;
#1701=EDGE_CURVE ( 'NONE', #5403, #7101, #18232, .T. ) ;
#1706=CARTESIAN_POINT ( 'NONE',  ( -1.461580736456473906, 65.46158073645646880, 48.05000000109247082 ) ) ;
#1716=CARTESIAN_POINT ( 'NONE',  ( -2.500000000000000888, 62.96446609406726935, 47.75000000218494023 ) ) ;
#1720=CARTESIAN_POINT ( 'NONE',  ( -2.066987300000001415, 64.00000000000000000, 44.95000000109246940 ) ) ;
#1726=CARTESIAN_POINT ( 'NONE',  ( -1.265664690411616068E-16, 66.06698730000000808, 48.75000000109246656 ) ) ;
#1743=DIRECTION ( 'NONE',  ( 0.000000000000000000, -1.000000000000000000, 0.000000000000000000 ) ) ;
#1746=CARTESIAN_POINT ( 'NONE',  ( 2.066987300000002303, 63.14382582708705627, 48.30000000109247082 ) ) ;
#1763=ORIENTED_EDGE ( 'NONE', *, *, #9342, .F. ) ;
#1771=CARTESIAN_POINT ( 'NONE',  ( 0.8561741729129460632, 66.06698730000000808, 48.50000000109246656 ) ) ;
#1772=FACE_OUTER_BOUND ( 'NONE', #8326, .T. ) ;
#1784=LINE ( 'NONE', #13730, #2855 ) ;
#1787=CARTESIAN_POINT ( 'NONE',  ( -2.500000000000001776, 64.00000000000000000, 48.39999999999999858 ) ) ;
#1791=AXIS2_PLACEMENT_3D ( 'NONE', #13713, #4815, #7646 ) ;
#1803=MECHANICAL_DESIGN_GEOMETRIC_PRESENTATION_REPRESENTATION('',(#7753),#12112);
#1806=CARTESIAN_POINT ( 'NONE',  ( 0.000000000000000000, 47.00000000000000711, -50.00000000000000000 ) ) ;
#1808=CARTESIAN_POINT ( 'NONE',  ( 14.99999999999998579, 73.00000000000001421, 26.99999999999997158 ) ) ;
#1815=CARTESIAN_POINT ( 'NONE',  ( -2.500000000000000888, 62.96446609406726935, 46.15000000218493881 ) ) ;
#1824=CARTESIAN_POINT ( 'NONE',  ( -2.500000000000001776, 64.00000000000000000, 46.00000000000000000 ) ) ;
#1825=CARTESIAN_POINT ( 'NONE',  ( 2.066987300000001415, 64.00000000000000000, 49.35000000109246798 ) ) ;
#1833=ORIENTED_EDGE ( 'NONE', *, *, #14412, .F. ) ;
#1836=VERTEX_POINT ( 'NONE', #15760 ) ;
#1840=CARTESIAN_POINT ( 'NONE',  ( 0.8561741729129472844, 61.93301270000000613, 48.20000000109248361 ) ) ;
#1847=CARTESIAN_POINT ( 'NONE',  ( -2.283493650000001818, 64.00000000000000000, 49.42500000163870766 ) ) ;
#1850=EDGE_CURVE ( 'NONE', #8256, #18922, #16853, .T. ) ;
#1853=EDGE_CURVE ( 'NONE', #14031, #2469, #13897, .T. ) ;
#1856=ORIENTED_EDGE ( 'NONE', *, *, #12110, .T. ) ;
#1867=CARTESIAN_POINT ( 'NONE',  ( 0.8561741729129471734, 61.93301270000000613, 47.40000000109247225 ) ) ;
#1876=EDGE_CURVE ( 'NONE', #13296, #19221, #8123, .T. ) ;
#1887=CARTESIAN_POINT ( 'NONE',  ( 1.035533905932738197, 66.50000000000000000, 49.74999999999998579 ) ) ;
#1905=DIRECTION ( 'NONE',  ( 1.000000000000000000, 0.000000000000000000, 0.000000000000000000 ) ) ;
#1907=DIRECTION ( 'NONE',  ( 0.000000000000000000, 0.000000000000000000, -1.000000000000000000 ) ) ;
#1910=LINE ( 'NONE', #4658, #1118 ) ;
#1912=ORIENTED_EDGE ( 'NONE', *, *, #10203, .T. ) ;
#1916=CARTESIAN_POINT ( 'NONE',  ( 1.035533905932738197, 66.50000000000000000, 45.85000000218494165 ) ) ;
#1918=VECTOR ( 'NONE', #946, 1000.000000000000000 ) ;
#1923=CARTESIAN_POINT ( 'NONE',  ( -1.530808498934192803E-16, 66.50000000000000000, 44.30000000218494449 ) ) ;
#1925=FACE_OUTER_BOUND ( 'NONE', #17623, .T. ) ;
#1928=CARTESIAN_POINT ( 'NONE',  ( 0.8561741729129472844, 61.93301270000000613, 48.40000000109247225 ) ) ;
#1942=EDGE_CURVE ( 'NONE', #18922, #13196, #12525, .T. ) ;
#1945=CARTESIAN_POINT ( 'NONE',  ( 0.8561741729129460632, 66.06698729999999387, 47.70000000109248361 ) ) ;
#1952=ADVANCED_FACE ( 'NONE', ( #14095 ), #6654, .T. ) ;
#1966=CARTESIAN_POINT ( 'NONE',  ( 3.796994071234847710E-16, 61.93301269999999903, 48.15000000109247225 ) ) ;
#1968=ORIENTED_EDGE ( 'NONE', *, *, #14647, .F. ) ;
#1975=DIRECTION ( 'NONE',  ( 0.000000000000000000, 0.000000000000000000, 1.000000000000000000 ) ) ;
#1976=CARTESIAN_POINT ( 'NONE',  ( -1.035533905932738641, 66.50000000000000000, 46.64999999999999858 ) ) ;
#1988=EDGE_LOOP ( 'NONE', ( #16561, #406, #2501, #11462 ) ) ;
#1993=ORIENTED_EDGE ( 'NONE', *, *, #420, .F. ) ;
#1999=CARTESIAN_POINT ( 'NONE',  ( -1.265664690411616068E-16, 66.06698730000000808, 44.75000000109247367 ) ) ;
#2006=CARTESIAN_POINT ( 'NONE',  ( 1.767766952966370653, 62.23223304703363112, 44.80000000218493739 ) ) ;
#2016=CARTESIAN_POINT ( 'NONE',  ( 2.066987300000002303, 63.14382582708705627, 47.70000000109247651 ) ) ;
#2017=CARTESIAN_POINT ( 'NONE',  ( -1.035533905932738863, 61.50000000000000000, 49.35000000000000853 ) ) ;
#2021=DIRECTION ( 'NONE',  ( -0.000000000000000000, 1.000000000000000000, -0.000000000000000000 ) ) ;
#2032=CARTESIAN_POINT ( 'NONE',  ( 0.8561741729129472844, 61.93301270000000613, 46.60000000109246088 ) ) ;
#2045=ORIENTED_EDGE ( 'NONE', *, *, #13819, .T. ) ;
#2058=CARTESIAN_POINT ( 'NONE',  ( 2.066987300000001859, 63.14382582708704916, 48.30000000109247082 ) ) ;
#2069=PLANE ( 'NONE',  #8114 ) ;
#2084=EDGE_LOOP ( 'NONE', ( #9328, #14077, #5381, #1326 ) ) ;
#2086=VECTOR ( 'NONE', #18460, 1000.000000000000000 ) ;
#2088=EDGE_CURVE ( 'NONE', #3058, #16441, #8492, .T. ) ;
#2090=DIRECTION ( 'NONE',  ( -0.000000000000000000, -1.000000000000000000, -0.000000000000000000 ) ) ;
#2095=CARTESIAN_POINT ( 'NONE',  ( 4.592425496802577917E-16, 61.50000000000000000, 46.19999999999999574 ) ) ;
#2103=DIRECTION ( 'NONE',  ( 0.000000000000000000, 0.000000000000000000, 1.000000000000000000 ) ) ;
#2105=ORIENTED_EDGE ( 'NONE', *, *, #7810, .T. ) ;
#2108=CARTESIAN_POINT ( 'NONE',  ( -1.035533905932738641, 66.50000000000000000, 46.75000000218494733 ) ) ;
#2117=CARTESIAN_POINT ( 'NONE',  ( -2.500000000000001776, 64.00000000000000000, 48.39999999999999858 ) ) ;
#2122=LINE ( 'NONE', #11210, #17713 ) ;
#2123=( BOUNDED_CURVE ( )  B_SPLINE_CURVE ( 2, ( #18705, #9940, #5551, #15758, #11415, #5647, #17499, #2319, #1038 ),
 .UNSPECIFIED., .F., .F. ) 
 B_SPLINE_CURVE_WITH_KNOTS ( ( 3, 2, 2, 2, 3 ),
 ( 0.6428571428571429047, 0.6607142857142856984, 0.6785714285714286031, 0.6964285714285712858, 0.7142857142857141906 ),
 .UNSPECIFIED. ) 
 CURVE ( )  GEOMETRIC_REPRESENTATION_ITEM ( )  RATIONAL_B_SPLINE_CURVE ( ( 1.000000000000000000, 0.9238795325112867385, 1.000000000000000000, 0.9238795325112867385, 1.000000000000000000, 0.9238795325112867385, 1.000000000000000000, 0.9238795325112871826, 0.9999999999999995559 ) ) 
 REPRESENTATION_ITEM ( '' )  );
#2124=EDGE_LOOP ( 'NONE', ( #2728, #6832, #19211, #11058 ) ) ;
#2130=CARTESIAN_POINT ( 'NONE',  ( 1.461580736456473684, 65.46158073645646880, 47.65000000109247225 ) ) ;
#2134=DIRECTION ( 'NONE',  ( 0.000000000000000000, 1.000000000000000000, 0.000000000000000000 ) ) ;
#2151=CARTESIAN_POINT ( 'NONE',  ( -1.767766952966370209, 65.76776695296638309, 47.49999999999999289 ) ) ;
#2154=EDGE_LOOP ( 'NONE', ( #4620, #3031, #1261, #11245 ) ) ;
#2161=CARTESIAN_POINT ( 'NONE',  ( -2.500000000000001776, 64.00000000000000000, 45.19999999999999574 ) ) ;
#2175=ADVANCED_FACE ( 'NONE', ( #16633 ), #15159, .F. ) ;
#2196=CARTESIAN_POINT ( 'NONE',  ( 1.767766952966369987, 65.76776695296638309, 45.80000000218493739 ) ) ;
#2207=DIRECTION ( 'NONE',  ( 1.000000000000000000, 0.000000000000000000, 0.000000000000000000 ) ) ;
#2209=CARTESIAN_POINT ( 'NONE',  ( -0.8561741729129461742, 66.06698729999999387, 45.60000000109246088 ) ) ;
#2219=CARTESIAN_POINT ( 'NONE',  ( -2.066987300000001415, 64.00000000000000000, 46.35000000109246798 ) ) ;
#2226=CARTESIAN_POINT ( 'NONE',  ( -2.066987300000001859, 64.85617417291294373, 47.90000000109247225 ) ) ;
#2235=CARTESIAN_POINT ( 'NONE',  ( 1.035533905932739751, 61.50000000000000000, 47.85000000000000142 ) ) ;
#2250=PLANE ( 'NONE',  #19151 ) ;
#2253=EDGE_LOOP ( 'NONE', ( #7371, #17666, #6169, #5889 ) ) ;
#2265=CARTESIAN_POINT ( 'NONE',  ( 32.50000000000000000, 52.00000000000000711, 12.50000000000000000 ) ) ;
#2276=CARTESIAN_POINT ( 'NONE',  ( -2.500000000000001776, 64.00000000000000000, 45.19999999999999574 ) ) ;
#2284=CARTESIAN_POINT ( 'NONE',  ( 1.035533905932738197, 66.50000000000000000, 45.85000000218494165 ) ) ;
#2291=CARTESIAN_POINT ( 'NONE',  ( 3.796994071234847710E-16, 61.93301269999999903, 47.35000000109246798 ) ) ;
#2302=CARTESIAN_POINT ( 'NONE',  ( -2.500000000000000888, 62.96446609406726935, 48.44999999999999574 ) ) ;
#2303=CARTESIAN_POINT ( 'NONE',  ( -1.265664690411616068E-16, 66.06698730000000808, 49.55000000109247082 ) ) ;
#2308=VERTEX_POINT ( 'NONE', #4381 ) ;
#2311=CARTESIAN_POINT ( 'NONE',  ( -2.066987300000000971, 63.14382582708704916, 45.60000000109246798 ) ) ;
#2316=CARTESIAN_POINT ( 'NONE',  ( -1.265664690411616068E-16, 66.06698730000000808, 46.15000000109247225 ) ) ;
#2319=CARTESIAN_POINT ( 'NONE',  ( -2.499999999999996003, 62.96446609406726225, 45.35000000218493454 ) ) ;
#2336=EDGE_CURVE ( 'NONE', #15781, #15589, #16730, .T. ) ;
#2342=PLANE ( 'NONE',  #1573 ) ;
#2361=CARTESIAN_POINT ( 'NONE',  ( 0.000000000000000000, 52.00000000000000711, 30.00000000000000000 ) ) ;
#2364=CARTESIAN_POINT ( 'NONE',  ( 1.767766952966370653, 62.23223304703363112, 45.50000000000000000 ) ) ;
#2368=FILL_AREA_STYLE_COLOUR ( '', #5648 ) ;
#2372=ORIENTED_EDGE ( 'NONE', *, *, #6725, .F. ) ;
#2377=CARTESIAN_POINT ( 'NONE',  ( -15.00000000000000000, -0.000000000000000000, 30.00000000000000000 ) ) ;
#2379=PLANE ( 'NONE',  #11132 ) ;
#2384=CARTESIAN_POINT ( 'NONE',  ( -2.066987300000001859, 64.85617417291294373, 49.50000000109246656 ) ) ;
#2389=AXIS2_PLACEMENT_3D ( 'NONE', #1499, #23, #1599 ) ;
#2393=CARTESIAN_POINT ( 'NONE',  ( -2.500000000000001776, 65.03553390593273775, 49.14999999999999858 ) ) ;
#2402=CARTESIAN_POINT ( 'NONE',  ( 0.8561741729129471734, 61.93301270000000613, 46.60000000109246798 ) ) ;
#2406=CARTESIAN_POINT ( 'NONE',  ( 0.8561741729129460632, 66.06698729999999387, 47.90000000109247225 ) ) ;
#2412=CARTESIAN_POINT ( 'NONE',  ( -1.767766952966369765, 62.23223304703363112, 47.69999999999999574 ) ) ;
#2426=CARTESIAN_POINT ( 'NONE',  ( 4.000000000000003553, 47.00000000000000711, 34.99999999999999289 ) ) ;
#2435=ORIENTED_EDGE ( 'NONE', *, *, #17847, .T. ) ;
#2436=DIRECTION ( 'NONE',  ( -1.000000000000000000, 0.000000000000000000, 0.000000000000000000 ) ) ;
#2469=VERTEX_POINT ( 'NONE', #16828 ) ;
#2473=EDGE_CURVE ( 'NONE', #3001, #7027, #9617, .T. ) ;
#2474=CARTESIAN_POINT ( 'NONE',  ( 3.796994071234847710E-16, 61.93301269999999903, 48.15000000109247225 ) ) ;
#2477=CARTESIAN_POINT ( 'NONE',  ( 1.035533905932739751, 61.50000000000000000, 46.35000000218494165 ) ) ;
#2484=CARTESIAN_POINT ( 'NONE',  ( -1.035533905932738641, 66.50000000000000000, 49.04999999999999716 ) ) ;
#2493=CARTESIAN_POINT ( 'NONE',  ( 3.796994071234847710E-16, 61.93301269999999903, 44.95000000109246940 ) ) ;
#2500=CARTESIAN_POINT ( 'NONE',  ( -1.265664690411616068E-16, 66.06698730000000808, 49.55000000109247082 ) ) ;
#2501=ORIENTED_EDGE ( 'NONE', *, *, #15791, .T. ) ;
#2508=CARTESIAN_POINT ( 'NONE',  ( -2.499999999999998668, 62.96446609406726225, 47.64999999999999858 ) ) ;
#2510=CARTESIAN_POINT ( 'NONE',  ( -1.767766952966369765, 62.23223304703363112, 48.49999999999999289 ) ) ;
#2517=SURFACE_STYLE_USAGE ( .BOTH. , #9774 ) ;
#2528=EDGE_CURVE ( 'NONE', #3632, #7844, #3779, .T. ) ;
#2530=CARTESIAN_POINT ( 'NONE',  ( 2.500000000000001776, 64.00000000000000000, 49.99999999999999289 ) ) ;
#2536=CARTESIAN_POINT ( 'NONE',  ( 14.99999999999998579, 52.00000000000000711, 23.99999999999997158 ) ) ;
#2559=VERTEX_POINT ( 'NONE', #7000 ) ;
#2563=CARTESIAN_POINT ( 'NONE',  ( -1.035533905932738863, 61.50000000000000000, 47.85000000218494165 ) ) ;
#2573=CARTESIAN_POINT ( 'NONE',  ( 2.066987300000001415, 64.00000000000000000, 48.35000000109246798 ) ) ;
#2584=CARTESIAN_POINT ( 'NONE',  ( 1.035533905932738197, 66.50000000000000000, 46.54999999999999716 ) ) ;
#2592=CARTESIAN_POINT ( 'NONE',  ( 2.066987300000001859, 63.14382582708704916, 45.10000000109246798 ) ) ;
#2594=EDGE_CURVE ( 'NONE', #11453, #15669, #18162, .T. ) ;
#2597=CARTESIAN_POINT ( 'NONE',  ( 2.066987300000001859, 64.85617417291294373, 48.60000000109246798 ) ) ;
#2622=EDGE_LOOP ( 'NONE', ( #14006, #10142 ) ) ;
#2628=CARTESIAN_POINT ( 'NONE',  ( 4.592425496802577917E-16, 61.50000000000000000, 47.10000000218494165 ) ) ;
#2646=SURFACE_SIDE_STYLE ('',( #4135 ) ) ;
#2668=CARTESIAN_POINT ( 'NONE',  ( -2.066987300000001415, 63.14382582708705627, 48.80000000109247082 ) ) ;
#2680=CARTESIAN_POINT ( 'NONE',  ( 2.500000000000002220, 62.96446609406726935, 47.14999999999999858 ) ) ;
#2682=EDGE_CURVE ( 'NONE', #14781, #19196, #15328, .T. ) ;
#2683=VECTOR ( 'NONE', #14243, 1000.000000000000000 ) ;
#2686=CARTESIAN_POINT ( 'NONE',  ( 1.767766952966370653, 62.23223304703363112, 48.80000000218494449 ) ) ;
#2697=CARTESIAN_POINT ( 'NONE',  ( -0.8561741729129461742, 66.06698729999999387, 49.60000000109246798 ) ) ;
#2714=VERTEX_POINT ( 'NONE', #8917 ) ;
#2728=ORIENTED_EDGE ( 'NONE', *, *, #1850, .F. ) ;
#2738=ORIENTED_EDGE ( 'NONE', *, *, #11216, .F. ) ;
#2740=( BOUNDED_CURVE ( )  B_SPLINE_CURVE ( 2, ( #11887, #17884, #13255, #10411, #19254, #2970, #14123, #3441, #2161 ),
 .UNSPECIFIED., .F., .F. ) 
 B_SPLINE_CURVE_WITH_KNOTS ( ( 3, 2, 2, 2, 3 ),
 ( 0.7857142857142856984, 0.8035714285714286031, 0.8214285714285713969, 0.8392857142857141906, 0.8571428571428569843 ),
 .UNSPECIFIED. ) 
 CURVE ( )  GEOMETRIC_REPRESENTATION_ITEM ( )  RATIONAL_B_SPLINE_CURVE ( ( 1.000000000000000000, 0.9238795325112867385, 1.000000000000000000, 0.9238795325112867385, 1.000000000000000000, 0.9238795325112867385, 1.000000000000000000, 0.9238795325112871826, 0.9999999999999995559 ) ) 
 REPRESENTATION_ITEM ( '' )  );
#2741=ORIENTED_EDGE ( 'NONE', *, *, #4371, .F. ) ;
#2753=LINE ( 'NONE', #1000, #7231 ) ;
#2764=CARTESIAN_POINT ( 'NONE',  ( 3.796994071234847710E-16, 61.93301269999999903, 44.95000000109246940 ) ) ;
#2766=AXIS2_PLACEMENT_3D ( 'NONE', #14766, #1435, #3200 ) ;
#2771=EDGE_CURVE ( 'NONE', #13230, #16897, #9705, .T. ) ;
#2773=CARTESIAN_POINT ( 'NONE',  ( -32.50000000000000000, 47.00000000000000711, -32.50000000000000000 ) ) ;
#2776=CARTESIAN_POINT ( 'NONE',  ( 2.500000000000002220, 62.96446609406726935, 47.94999999999999574 ) ) ;
#2777=CARTESIAN_POINT ( 'NONE',  ( 2.066987300000001415, 64.85617417291294373, 47.80000000109247082 ) ) ;
#2783=ORIENTED_EDGE ( 'NONE', *, *, #19177, .T. ) ;
#2784=EDGE_CURVE ( 'NONE', #4943, #18801, #6593, .T. ) ;
#2788=FACE_OUTER_BOUND ( 'NONE', #6329, .T. ) ;
#2789=ADVANCED_FACE ( 'NONE', ( #1772 ), #11848, .T. ) ;
#2792=CARTESIAN_POINT ( 'NONE',  ( -2.066987300000001415, 63.14382582708705627, 44.80000000109247082 ) ) ;
#2803=PLANE ( 'NONE',  #5988 ) ;
#2816=AXIS2_PLACEMENT_3D ( 'NONE', #12177, #127, #12077 ) ;
#2824=CARTESIAN_POINT ( 'NONE',  ( 1.767766952966369987, 65.76776695296638309, 45.69999999999999574 ) ) ;
#2831=DIRECTION ( 'NONE',  ( -0.000000000000000000, -0.000000000000000000, -1.000000000000000000 ) ) ;
#2834=EDGE_LOOP ( 'NONE', ( #955, #34 ) ) ;
#2839=ORIENTED_EDGE ( 'NONE', *, *, #18941, .T. ) ;
#2850=PRODUCT ( 'Spring-Loaded Carriage Elevator Arm', 'Spring-Loaded Carriage Elevator Arm', '', ( #2952 ) ) ;
#2852=DIRECTION ( 'NONE',  ( -0.000000000000000000, 1.000000000000000000, -0.000000000000000000 ) ) ;
#2855=VECTOR ( 'NONE', #311, 1000.000000000000000 ) ;
#2862=CARTESIAN_POINT ( 'NONE',  ( -15.00000000000000000, 49.99999999999997158, -4.956352788505161414E-14 ) ) ;
#2867=CARTESIAN_POINT ( 'NONE',  ( 2.066987300000001859, 64.85617417291294373, 46.00000000109246656 ) ) ;
#2869=VECTOR ( 'NONE', #8507, 1000.000000000000000 ) ;
#2879=CARTESIAN_POINT ( 'NONE',  ( -2.500000000000001776, 65.03553390593273775, 47.54999999999999716 ) ) ;
#2880=CARTESIAN_POINT ( 'NONE',  ( -0.8561741729129461742, 66.06698730000000808, 45.60000000109246798 ) ) ;
#2892=CARTESIAN_POINT ( 'NONE',  ( -1.530808498934192803E-16, 66.50000000000000000, 47.50000000218494023 ) ) ;
#2915=CARTESIAN_POINT ( 'NONE',  ( -10.00000000000000000, 0.000000000000000000, 0.000000000000000000 ) ) ;
#2921=CARTESIAN_POINT ( 'NONE',  ( 2.500000000000001776, 64.00000000000000000, 47.19999999999999574 ) ) ;
#2922=CARTESIAN_POINT ( 'NONE',  ( -41.00000000000000000, 47.00000000000000711, -67.72004514666936359 ) ) ;
#2932=ORIENTED_EDGE ( 'NONE', *, *, #19177, .F. ) ;
#2938=VERTEX_POINT ( 'NONE', #11156 ) ;
#2947=ORIENTED_EDGE ( 'NONE', *, *, #7881, .T. ) ;
#2948=EDGE_CURVE ( 'NONE', #15781, #8882, #6477, .T. ) ;
#2952=PRODUCT_CONTEXT ( 'NONE', #10703, 'mechanical' ) ;
#2961=CARTESIAN_POINT ( 'NONE',  ( -2.066987300000001415, 64.00000000000000000, 46.35000000109246798 ) ) ;
#2967=ORIENTED_EDGE ( 'NONE', *, *, #57, .T. ) ;
#2968=CARTESIAN_POINT ( 'NONE',  ( -10.00000000000000000, 50.00000000000000711, 37.00000000000000000 ) ) ;
#2970=CARTESIAN_POINT ( 'NONE',  ( -1.035533905932738863, 61.50000000000000000, 45.34999999999998721 ) ) ;
#2971=( BOUNDED_CURVE ( )  B_SPLINE_CURVE ( 2, ( #11661, #5892, #10282, #16179, #16381 ),
 .UNSPECIFIED., .F., .F. ) 
 B_SPLINE_CURVE_WITH_KNOTS ( ( 3, 2, 3 ),
 ( 0.8571428571428568732, 0.8749999999999998890, 0.8928571428571429047 ),
 .UNSPECIFIED. ) 
 CURVE ( )  GEOMETRIC_REPRESENTATION_ITEM ( )  RATIONAL_B_SPLINE_CURVE ( ( 1.000000000000000888, 0.9238795325112857393, 1.000000000000000000, 0.9238795325112867385, 1.000000000000000000 ) ) 
 REPRESENTATION_ITEM ( '' )  );
#2974=CARTESIAN_POINT ( 'NONE',  ( -2.066987300000000971, 63.14382582708704916, 47.40000000109247225 ) ) ;
#2978=PRODUCT_DEFINITION_FORMATION_WITH_SPECIFIED_SOURCE ( 'ANY', '', #2850, .NOT_KNOWN. ) ;
#2985=CARTESIAN_POINT ( 'NONE',  ( -2.066987300000001415, 63.14382582708705627, 46.60000000109246088 ) ) ;
#2998=ADVANCED_FACE ( 'NONE', ( #400 ), #14012, .F. ) ;
#2999=CARTESIAN_POINT ( 'NONE',  ( 1.767766952966370653, 62.23223304703363112, 44.80000000218493739 ) ) ;
#3000=ORIENTED_EDGE ( 'NONE', *, *, #2473, .F. ) ;
#3001=VERTEX_POINT ( 'NONE', #18344 ) ;
#3014=CARTESIAN_POINT ( 'NONE',  ( -2.066987300000001859, 64.85617417291294373, 49.50000000109246656 ) ) ;
#3026=CIRCLE ( 'NONE', #13984, 2.999999999999999112 ) ;
#3031=ORIENTED_EDGE ( 'NONE', *, *, #12037, .T. ) ;
#3045=LINE ( 'NONE', #9019, #4094 ) ;
#3054=CARTESIAN_POINT ( 'NONE',  ( -1.767766952966370209, 65.76776695296638309, 48.29999999999999716 ) ) ;
#3058=VERTEX_POINT ( 'NONE', #16771 ) ;
#3062=EDGE_CURVE ( 'NONE', #3881, #13516, #17247, .T. ) ;
#3073=CARTESIAN_POINT ( 'NONE',  ( -1.265664690411616068E-16, 66.06698730000000808, 45.55000000109246372 ) ) ;
#3078=ORIENTED_EDGE ( 'NONE', *, *, #15657, .F. ) ;
#3082=CARTESIAN_POINT ( 'NONE',  ( 1.035533905932739751, 61.50000000000000000, 47.95000000218495018 ) ) ;
#3084=CARTESIAN_POINT ( 'NONE',  ( -0.8561741729129461742, 66.06698729999999387, 46.40000000109246514 ) ) ;
#3088=AXIS2_PLACEMENT_3D ( 'NONE', #17603, #19073, #19273 ) ;
#3112=VECTOR ( 'NONE', #11226, 1000.000000000000000 ) ;
#3113=CARTESIAN_POINT ( 'NONE',  ( 3.796994071234847710E-16, 61.93301269999999903, 48.15000000109247225 ) ) ;
#3128=ORIENTED_EDGE ( 'NONE', *, *, #8748, .F. ) ;
#3137=ADVANCED_FACE ( 'NONE', ( #7132 ), #2342, .T. ) ;
#3153=CIRCLE ( 'NONE', #6896, 2.499999999999998668 ) ;
#3161=DIRECTION ( 'NONE',  ( 0.000000000000000000, -1.000000000000000000, 0.000000000000000000 ) ) ;
#3169=AXIS2_PLACEMENT_3D ( 'NONE', #17657, #4232, #3849 ) ;
#3170=CYLINDRICAL_SURFACE ( 'NONE', #6872, 2.500000000000001776 ) ;
#3176=CARTESIAN_POINT ( 'NONE',  ( -1.461580736456473906, 65.46158073645646880, 46.45000000109246940 ) ) ;
#3181=CARTESIAN_POINT ( 'NONE',  ( -14.99999999999999645, 52.00000000000000711, 23.99999999999997868 ) ) ;
#3189=CARTESIAN_POINT ( 'NONE',  ( -1.035533905932738863, 61.50000000000000000, 47.85000000218494165 ) ) ;
#3191=CARTESIAN_POINT ( 'NONE',  ( -0.8561741729129465073, 61.93301270000000613, 46.70000000109248361 ) ) ;
#3198=B_SPLINE_CURVE_WITH_KNOTS ( 'NONE', 1,
 ( #13501, #5963 ),
 .UNSPECIFIED., .F., .F.,
 ( 2, 2 ),
 ( 0.000000000000000000, 1.000000000000000000 ),
 .UNSPECIFIED. ) ;
#3199=CARTESIAN_POINT ( 'NONE',  ( 1.461580736456473906, 62.53841926354353120, 46.85000000109246798 ) ) ;
#3200=DIRECTION ( 'NONE',  ( 1.000000000000000000, 0.000000000000000000, 0.000000000000000000 ) ) ;
#3218=CARTESIAN_POINT ( 'NONE',  ( -1.461580736456473462, 62.53841926354353120, 48.85000000109246798 ) ) ;
#3239=CARTESIAN_POINT ( 'NONE',  ( 1.461580736456473684, 65.46158073645646880, 49.25000000109246656 ) ) ;
#3241=ORIENTED_EDGE ( 'NONE', *, *, #7586, .T. ) ;
#3248=CARTESIAN_POINT ( 'NONE',  ( -2.500000000000001776, 65.03553390593273775, 46.74999999999999289 ) ) ;
#3267=( BOUNDED_CURVE ( )  B_SPLINE_CURVE ( 2, ( #4187, #1044, #2999, #19184, #10140, #7314, #7220, #11515, #5751 ),
 .UNSPECIFIED., .F., .F. ) 
 B_SPLINE_CURVE_WITH_KNOTS ( ( 3, 2, 2, 2, 3 ),
 ( 0.7857142857142856984, 0.8035714285714286031, 0.8214285714285712858, 0.8392857142857141906, 0.8571428571428568732 ),
 .UNSPECIFIED. ) 
 CURVE ( )  GEOMETRIC_REPRESENTATION_ITEM ( )  RATIONAL_B_SPLINE_CURVE ( ( 1.000000000000000000, 0.9238795325112867385, 1.000000000000000000, 0.9238795325112867385, 1.000000000000000000, 0.9238795325112867385, 1.000000000000000000, 0.9238795325112877377, 0.9999999999999990008 ) ) 
 REPRESENTATION_ITEM ( '' )  );
#3275=FACE_OUTER_BOUND ( 'NONE', #13101, .T. ) ;
#3286=CARTESIAN_POINT ( 'NONE',  ( -1.767766952966370209, 65.76776695296638309, 45.20000000218494307 ) ) ;
#3290=CARTESIAN_POINT ( 'NONE',  ( 3.796994071234847710E-16, 61.93301269999999903, 45.95000000109246940 ) ) ;
#3298=CARTESIAN_POINT ( 'NONE',  ( -1.461580736456473462, 62.53841926354353120, 49.05000000109247082 ) ) ;
#3300=DIRECTION ( 'NONE',  ( 1.000000000000000000, 0.000000000000000000, 0.000000000000000000 ) ) ;
#3305=ORIENTED_EDGE ( 'NONE', *, *, #11039, .T. ) ;
#3313=DIRECTION ( 'NONE',  ( -0.000000000000000000, 1.000000000000000000, -0.000000000000000000 ) ) ;
#3338=ADVANCED_FACE ( 'NONE', ( #13991 ), #18868, .F. ) ;
#3341=CARTESIAN_POINT ( 'NONE',  ( -0.8561741729129461742, 66.06698730000000808, 48.60000000109246798 ) ) ;
#3369=ORIENTED_EDGE ( 'NONE', *, *, #9870, .F. ) ;
#3380=CARTESIAN_POINT ( 'NONE',  ( -2.500000000000001776, 65.03553390593273775, 46.05000000218494449 ) ) ;
#3389=CARTESIAN_POINT ( 'NONE',  ( -2.066987300000001859, 64.85617417291294373, 47.30000000109247082 ) ) ;
#3406=CARTESIAN_POINT ( 'NONE',  ( -0.8561741729129461742, 66.06698729999999387, 47.00000000109247367 ) ) ;
#3411=DIRECTION ( 'NONE',  ( -0.000000000000000000, -1.000000000000000000, -0.000000000000000000 ) ) ;
#3420=ORIENTED_EDGE ( 'NONE', *, *, #2948, .F. ) ;
#3430=CARTESIAN_POINT ( 'NONE',  ( -1.461580736456473906, 65.46158073645646880, 47.05000000109247082 ) ) ;
#3438=ORIENTED_EDGE ( 'NONE', *, *, #5281, .F. ) ;
#3441=CARTESIAN_POINT ( 'NONE',  ( -2.499999999999996003, 62.96446609406726225, 45.25000000000000000 ) ) ;
#3446=AXIS2_PLACEMENT_3D ( 'NONE', #2536, #8518, #14493 ) ;
#3451=DIRECTION ( 'NONE',  ( -0.000000000000000000, -0.000000000000000000, -1.000000000000000000 ) ) ;
#3456=AXIS2_PLACEMENT_3D ( 'NONE', #12521, #274, #18123 ) ;
#3463=MECHANICAL_DESIGN_GEOMETRIC_PRESENTATION_REPRESENTATION('',(#7849),#355);
#3468=CARTESIAN_POINT ( 'NONE',  ( -1.767766952966370209, 65.76776695296638309, 46.00000000218494733 ) ) ;
#3469=AXIS2_PLACEMENT_3D ( 'NONE', #11925, #11718, #14779 ) ;
#3474=DIRECTION ( 'NONE',  ( -0.000000000000000000, -1.000000000000000000, -0.000000000000000000 ) ) ;
#3475=AXIS2_PLACEMENT_3D ( 'NONE', #18910, #12638, #8415 ) ;
#3479=CARTESIAN_POINT ( 'NONE',  ( 1.767766952966369987, 65.76776695296638309, 47.40000000218494591 ) ) ;
#3488=CARTESIAN_POINT ( 'NONE',  ( 3.796994071234847710E-16, 61.93301269999999903, 46.75000000109246656 ) ) ;
#3496=FACE_OUTER_BOUND ( 'NONE', #11086, .T. ) ;
#3497=( BOUNDED_CURVE ( )  B_SPLINE_CURVE ( 2, ( #10139, #14281, #3987, #12710, #3803, #9769, #2510, #9856, #8588 ),
 .UNSPECIFIED., .F., .F. ) 
 B_SPLINE_CURVE_WITH_KNOTS ( ( 3, 2, 2, 2, 3 ),
 ( 0.2142857142857141350, 0.2321428571428569565, 0.2499999999999997224, 0.2678571428571425161, 0.2857142857142853098 ),
 .UNSPECIFIED. ) 
 CURVE ( )  GEOMETRIC_REPRESENTATION_ITEM ( )  RATIONAL_B_SPLINE_CURVE ( ( 1.000000000000000666, 0.9238795325112861834, 1.000000000000000000, 0.9238795325112867385, 1.000000000000000000, 0.9238795325112867385, 1.000000000000000000, 0.9238795325112884038, 0.9999999999999983347 ) ) 
 REPRESENTATION_ITEM ( '' )  );
#3510=CARTESIAN_POINT ( 'NONE',  ( 3.796994071234847710E-16, 61.93301269999999903, 44.95000000109246940 ) ) ;
#3531=CARTESIAN_POINT ( 'NONE',  ( -1.265664690411616068E-16, 66.06698730000000808, 49.35000000109246798 ) ) ;
#3537=ADVANCED_FACE ( 'NONE', ( #1606 ), #7581, .T. ) ;
#3539=VERTEX_POINT ( 'NONE', #18075 ) ;
#3547=CARTESIAN_POINT ( 'NONE',  ( -2.500000000000001776, 64.00000000000000000, 49.30000000218494449 ) ) ;
#3551=ORIENTED_EDGE ( 'NONE', *, *, #387, .T. ) ;
#3563=CARTESIAN_POINT ( 'NONE',  ( 0.000000000000000000, 64.00000000000000000, 49.99999999999999289 ) ) ;
#3572=CARTESIAN_POINT ( 'NONE',  ( -2.500000000000001776, 64.00000000000000000, 46.10000000218494165 ) ) ;
#3580=CARTESIAN_POINT ( 'NONE',  ( 0.000000000000000000, 64.00000000000000000, 49.99999999999999289 ) ) ;
#3582=CARTESIAN_POINT ( 'NONE',  ( -0.8561741729129465073, 61.93301270000000613, 49.10000000109246088 ) ) ;
#3596=CARTESIAN_POINT ( 'NONE',  ( 3.796994071234847710E-16, 61.93301269999999903, 46.55000000109247082 ) ) ;
#3616=CARTESIAN_POINT ( 'NONE',  ( -14.99999999999999645, 52.00000000000000711, 26.99999999999997868 ) ) ;
#3623=CARTESIAN_POINT ( 'NONE',  ( -14.99999999999999645, 73.00000000000001421, 20.99999999999998224 ) ) ;
#3632=VERTEX_POINT ( 'NONE', #15428 ) ;
#3656=DIRECTION ( 'NONE',  ( 0.000000000000000000, 0.000000000000000000, 1.000000000000000000 ) ) ;
#3659=DIRECTION ( 'NONE',  ( -1.000000000000000000, -0.000000000000000000, -0.000000000000000000 ) ) ;
#3662=ADVANCED_FACE ( 'NONE', ( #15229 ), #6695, .F. ) ;
#3670=CARTESIAN_POINT ( 'NONE',  ( -2.500000000000001776, 64.00000000000000000, 44.50000000218494733 ) ) ;
#3679=CARTESIAN_POINT ( 'NONE',  ( 1.767766952966369987, 65.76776695296638309, 49.69999999999999574 ) ) ;
#3685=DIRECTION ( 'NONE',  ( -1.000000000000000000, 0.000000000000000000, 0.000000000000000000 ) ) ;
#3686=VERTEX_POINT ( 'NONE', #8352 ) ;
#3688=CARTESIAN_POINT ( 'NONE',  ( -0.8561741729129461742, 66.06698730000000808, 46.20000000109248361 ) ) ;
#3693=CARTESIAN_POINT ( 'NONE',  ( -2.066987300000001415, 63.14382582708705627, 46.40000000109246514 ) ) ;
#3695=VERTEX_POINT ( 'NONE', #9807 ) ;
#3710=VERTEX_POINT ( 'NONE', #10088 ) ;
#3717=VERTEX_POINT ( 'NONE', #9901 ) ;
#3734=ORIENTED_EDGE ( 'NONE', *, *, #11216, .T. ) ;
#3737=EDGE_CURVE ( 'NONE', #7027, #16441, #12251, .T. ) ;
#3741=MANIFOLD_SOLID_BREP ( 'Boss-Extrude5', #1016 ) ;
#3746=FILL_AREA_STYLE ('',( #2368 ) ) ;
#3750=EDGE_LOOP ( 'NONE', ( #9954, #17956, #8330, #10933 ) ) ;
#3755=EDGE_CURVE ( 'NONE', #1836, #292, #18844, .T. ) ;
#3758=DIRECTION ( 'NONE',  ( 0.000000000000000000, 0.000000000000000000, 1.000000000000000000 ) ) ;
#3766=CARTESIAN_POINT ( 'NONE',  ( -2.066987300000001859, 64.85617417291294373, 47.10000000109246798 ) ) ;
#3778=CARTESIAN_POINT ( 'NONE',  ( -1.530808498934192803E-16, 66.50000000000000000, 48.99999999999999289 ) ) ;
#3779=LINE ( 'NONE', #18773, #1198 ) ;
#3781=CARTESIAN_POINT ( 'NONE',  ( 2.500000000000001776, 64.00000000000000000, 48.90000000218494591 ) ) ;
#3782=ADVANCED_FACE ( 'NONE', ( #15710 ), #8628, .F. ) ;
#3789=CARTESIAN_POINT ( 'NONE',  ( -2.066987300000000971, 63.14382582708704916, 46.40000000109247225 ) ) ;
#3791=CYLINDRICAL_SURFACE ( 'NONE', #18227, 2.500000000000002220 ) ;
#3794=CARTESIAN_POINT ( 'NONE',  ( 1.461580736456473906, 62.53841926354353120, 45.85000000109246798 ) ) ;
#3803=CARTESIAN_POINT ( 'NONE',  ( 4.592425496802577917E-16, 61.50000000000000000, 48.59999999999999432 ) ) ;
#3808=FILL_AREA_STYLE_COLOUR ( '', #10541 ) ;
#3815=CARTESIAN_POINT ( 'NONE',  ( -2.500000000000001776, 64.00000000000000000, 47.59999999999999432 ) ) ;
#3848=CARTESIAN_POINT ( 'NONE',  ( -32.50000000000000000, 52.00000000000000711, 17.49999999999999645 ) ) ;
#3849=DIRECTION ( 'NONE',  ( 0.000000000000000000, 0.000000000000000000, 1.000000000000000000 ) ) ;
#3850=EDGE_CURVE ( 'NONE', #7747, #13196, #3045, .T. ) ;
#3859=CARTESIAN_POINT ( 'NONE',  ( -0.8561741729129465073, 61.93301270000000613, 48.90000000109247225 ) ) ;
#3861=FACE_BOUND ( 'NONE', #1383, .T. ) ;
#3867=CARTESIAN_POINT ( 'NONE',  ( -1.035533905932738863, 61.50000000000000000, 49.35000000000000142 ) ) ;
#3868=CARTESIAN_POINT ( 'NONE',  ( 3.796994071234847710E-16, 61.93301269999999903, 49.15000000109246514 ) ) ;
#3869=CARTESIAN_POINT ( 'NONE',  ( 4.592425496802577917E-16, 61.50000000000000000, 48.70000000218494307 ) ) ;
#3875=EDGE_CURVE ( 'NONE', #17639, #16538, #13617, .T. ) ;
#3880=CARTESIAN_POINT ( 'NONE',  ( -0.8561741729129461742, 66.06698729999999387, 48.00000000109246656 ) ) ;
#3881=VERTEX_POINT ( 'NONE', #16576 ) ;
#3899=VERTEX_POINT ( 'NONE', #208 ) ;
#3923=ORIENTED_EDGE ( 'NONE', *, *, #9342, .T. ) ;
#3933=ORIENTED_EDGE ( 'NONE', *, *, #18463, .T. ) ;
#3940=DIRECTION ( 'NONE',  ( -2.602085213965211135E-16, 1.000000000000000000, -0.000000000000000000 ) ) ;
#3941=EDGE_CURVE ( 'NONE', #3899, #13296, #2971, .T. ) ;
#3948=DIRECTION ( 'NONE',  ( 0.000000000000000000, 0.000000000000000000, -1.000000000000000000 ) ) ;
#3953=CARTESIAN_POINT ( 'NONE',  ( 0.8561741729129472844, 61.93301270000000613, 49.00000000109246656 ) ) ;
#3956=CARTESIAN_POINT ( 'NONE',  ( -2.499999999999992006, 62.96446609406726225, 46.15000000218496012 ) ) ;
#3965=CARTESIAN_POINT ( 'NONE',  ( -1.035533905932738641, 66.50000000000000000, 49.85000000000000142 ) ) ;
#3967=EDGE_CURVE ( 'NONE', #16382, #13196, #18547, .T. ) ;
#3975=CARTESIAN_POINT ( 'NONE',  ( 1.461580736456473684, 65.46158073645646880, 45.25000000109247367 ) ) ;
#3979=CARTESIAN_POINT ( 'NONE',  ( -1.461580736456473906, 65.46158073645646880, 49.65000000109246514 ) ) ;
#3987=CARTESIAN_POINT ( 'NONE',  ( 1.767766952966370653, 62.23223304703363112, 48.69999999999999574 ) ) ;
#3993=( NAMED_UNIT ( * ) SI_UNIT ( $, .STERADIAN. ) SOLID_ANGLE_UNIT ( ) );
#4019=DIRECTION ( 'NONE',  ( -0.000000000000000000, -0.000000000000000000, -1.000000000000000000 ) ) ;
#4020=EDGE_LOOP ( 'NONE', ( #15496, #14883, #8830, #14322, #17070, #15793 ) ) ;
#4022=CARTESIAN_POINT ( 'NONE',  ( 2.500000000000001776, 64.00000000000000000, 45.59999999999999432 ) ) ;
#4023=ORIENTED_EDGE ( 'NONE', *, *, #8655, .T. ) ;
#4025=DIRECTION ( 'NONE',  ( 1.000000000000000000, 0.000000000000000000, 0.000000000000000000 ) ) ;
#4033=CARTESIAN_POINT ( 'NONE',  ( 1.035533905932739751, 61.50000000000000000, 47.95000000218494307 ) ) ;
#4040=CARTESIAN_POINT ( 'NONE',  ( -4.000000000000001776, 67.00000000000000000, 30.00000000000000000 ) ) ;
#4045=CARTESIAN_POINT ( 'NONE',  ( -0.8561741729129465073, 61.93301270000000613, 47.30000000109247082 ) ) ;
#4049=DIRECTION ( 'NONE',  ( 0.000000000000000000, -0.000000000000000000, -1.000000000000000000 ) ) ;
#4058=CARTESIAN_POINT ( 'NONE',  ( -2.500000000000001776, 65.03553390593273775, 49.95000000000000284 ) ) ;
#4059=CARTESIAN_POINT ( 'NONE',  ( 0.8561741729129471734, 61.93301270000000613, 49.20000000109247651 ) ) ;
#4066=CARTESIAN_POINT ( 'NONE',  ( -0.8561741729129461742, 66.06698730000000808, 45.40000000109247225 ) ) ;
#4069=CARTESIAN_POINT ( 'NONE',  ( 32.50000000000000000, 52.00000000000000711, -35.00000000000000000 ) ) ;
#4073=CARTESIAN_POINT ( 'NONE',  ( -2.066987300000001415, 63.14382582708705627, 47.40000000109247225 ) ) ;
#4082=CARTESIAN_POINT ( 'NONE',  ( 1.767766952966370653, 62.23223304703363112, 47.89999999999999858 ) ) ;
#4093=ORIENTED_EDGE ( 'NONE', *, *, #18614, .T. ) ;
#4094=VECTOR ( 'NONE', #1583, 1000.000000000000000 ) ;
#4117=AXIS2_PLACEMENT_3D ( 'NONE', #5748, #16336, #16429 ) ;
#4119=CARTESIAN_POINT ( 'NONE',  ( 2.500000000000001776, 64.00000000000000000, 46.39999999999999858 ) ) ;
#4135=SURFACE_STYLE_FILL_AREA ( #3746 ) ;
#4151=ADVANCED_FACE ( 'NONE', ( #5289 ), #9785, .F. ) ;
#4155=CARTESIAN_POINT ( 'NONE',  ( 2.066987300000001415, 64.00000000000000000, 46.75000000109247367 ) ) ;
#4163=CARTESIAN_POINT ( 'NONE',  ( -15.00000000000000000, 50.00000000000000711, 37.00000000000000000 ) ) ;
#4166=CARTESIAN_POINT ( 'NONE',  ( 1.035533905932739751, 61.50000000000000000, 47.85000000000000142 ) ) ;
#4178=CARTESIAN_POINT ( 'NONE',  ( -0.8561741729129465073, 61.93301270000000613, 48.30000000109247082 ) ) ;
#4187=CARTESIAN_POINT ( 'NONE',  ( 2.500000000000001776, 64.00000000000000000, 44.90000000218493881 ) ) ;
#4188=ORIENTED_EDGE ( 'NONE', *, *, #16499, .F. ) ;
#4189=ORIENTED_EDGE ( 'NONE', *, *, #4915, .T. ) ;
#4207=LINE ( 'NONE', #10160, #7489 ) ;
#4211=CARTESIAN_POINT ( 'NONE',  ( -10.00000000000000000, 35.00000000000000000, 37.00000000000000000 ) ) ;
#4215=VERTEX_POINT ( 'NONE', #11347 ) ;
#4218=ORIENTED_EDGE ( 'NONE', *, *, #19229, .F. ) ;
#4230=CARTESIAN_POINT ( 'NONE',  ( 32.50000000000000000, 52.00000000000000711, -37.50000000000000711 ) ) ;
#4232=DIRECTION ( 'NONE',  ( -0.000000000000000000, -1.000000000000000000, -0.000000000000000000 ) ) ;
#4238=EDGE_CURVE ( 'NONE', #16538, #10567, #18817, .T. ) ;
#4247=VECTOR ( 'NONE', #7524, 1000.000000000000000 ) ;
#4248=CARTESIAN_POINT ( 'NONE',  ( -2.066987300000001859, 64.85617417291294373, 46.30000000109247082 ) ) ;
#4259=CARTESIAN_POINT ( 'NONE',  ( 2.500000000000001776, 64.00000000000000000, 47.19999999999999574 ) ) ;
#4260=CARTESIAN_POINT ( 'NONE',  ( 3.796994071234847710E-16, 61.93301269999999903, 45.95000000109246940 ) ) ;
#4263=VECTOR ( 'NONE', #3474, 1000.000000000000000 ) ;
#4271=CARTESIAN_POINT ( 'NONE',  ( -1.767766952966370209, 65.76776695296638309, 49.20000000218494307 ) ) ;
#4273=CIRCLE ( 'NONE', #15542, 2.499999999999998668 ) ;
#4274=VECTOR ( 'NONE', #13780, 1000.000000000000000 ) ;
#4275=CARTESIAN_POINT ( 'NONE',  ( -0.8561741729129465073, 61.93301270000000613, 47.50000000109246656 ) ) ;
#4284=CARTESIAN_POINT ( 'NONE',  ( -10.00000000000000000, 47.00000000000000711, 0.000000000000000000 ) ) ;
#4286=VECTOR ( 'NONE', #14546, 1000.000000000000000 ) ;
#4316=CARTESIAN_POINT ( 'NONE',  ( 2.500000000000001776, 64.00000000000000000, 49.99999999999999289 ) ) ;
#4324=CARTESIAN_POINT ( 'NONE',  ( 2.500000000000001776, 65.03553390593273775, 47.35000000218494165 ) ) ;
#4326=LINE ( 'NONE', #10284, #12826 ) ;
#4332=DIRECTION ( 'NONE',  ( 2.602085213965211135E-16, -1.000000000000000000, 0.000000000000000000 ) ) ;
#4339=FACE_OUTER_BOUND ( 'NONE', #7454, .T. ) ;
#4344=CARTESIAN_POINT ( 'NONE',  ( -2.066987300000001415, 64.00000000000000000, 45.55000000109246372 ) ) ;
#4349=EDGE_CURVE ( 'NONE', #10567, #13006, #17626, .T. ) ;
#4359=CARTESIAN_POINT ( 'NONE',  ( 4.592425496802577917E-16, 61.50000000000000000, 47.79999999999999716 ) ) ;
#4360=CARTESIAN_POINT ( 'NONE',  ( 1.461580736456473906, 62.53841926354353120, 46.05000000109246372 ) ) ;
#4368=CARTESIAN_POINT ( 'NONE',  ( -1.767766952966370209, 65.76776695296638309, 48.40000000218494591 ) ) ;
#4371=EDGE_CURVE ( 'NONE', #17355, #8256, #8996, .T. ) ;
#4381=CARTESIAN_POINT ( 'NONE',  ( -10.00000000000000000, 35.00000000000000000, 33.99999999999999289 ) ) ;
#4387=EDGE_LOOP ( 'NONE', ( #16049, #4801, #18434, #10063 ) ) ;
#4427=VERTEX_POINT ( 'NONE', #12426 ) ;
#4449=ADVANCED_FACE ( 'NONE', ( #6364 ), #15275, .T. ) ;
#4456=DIRECTION ( 'NONE',  ( -1.000000000000000000, 0.000000000000000000, -0.000000000000000000 ) ) ;
#4462=CARTESIAN_POINT ( 'NONE',  ( -2.066987300000000971, 63.14382582708704916, 45.80000000109246372 ) ) ;
#4463=ADVANCED_FACE ( 'NONE', ( #15469 ), #6261, .F. ) ;
#4475=CARTESIAN_POINT ( 'NONE',  ( 1.461580736456473684, 65.46158073645646880, 45.45000000109246940 ) ) ;
#4500=ORIENTED_EDGE ( 'NONE', *, *, #9137, .F. ) ;
#4503=DIRECTION ( 'NONE',  ( 0.000000000000000000, 0.000000000000000000, 1.000000000000000000 ) ) ;
#4506=CARTESIAN_POINT ( 'NONE',  ( -41.00000000000000000, 47.00000000000000711, -50.00000000000000000 ) ) ;
#4510=CARTESIAN_POINT ( 'NONE',  ( 32.50000000000000000, 52.00000000000000711, 15.00000000000000000 ) ) ;
#4531=( BOUNDED_CURVE ( )  B_SPLINE_CURVE ( 2, ( #3547, #7870, #505, #6492, #13837, #4930, #10887, #16881, #7664 ),
 .UNSPECIFIED., .F., .F. ) 
 B_SPLINE_CURVE_WITH_KNOTS ( ( 3, 2, 2, 2, 3 ),
 ( 0.000000000000000000, 0.01785714285714289085, 0.03571428571428578169, 0.05357142857142867254, 0.07142857142857156338 ),
 .UNSPECIFIED. ) 
 CURVE ( )  GEOMETRIC_REPRESENTATION_ITEM ( )  RATIONAL_B_SPLINE_CURVE ( ( 1.000000000000000000, 0.9238795325112867385, 1.000000000000000000, 0.9238795325112867385, 1.000000000000000000, 0.9238795325112867385, 1.000000000000000000, 0.9238795325112861834, 1.000000000000000666 ) ) 
 REPRESENTATION_ITEM ( '' )  );
#4543=CARTESIAN_POINT ( 'NONE',  ( 1.461580736456473906, 62.53841926354353120, 45.85000000109246798 ) ) ;
#4547=ORIENTED_EDGE ( 'NONE', *, *, #12722, .T. ) ;
#4557=CARTESIAN_POINT ( 'NONE',  ( -0.8561741729129461742, 66.06698730000000808, 47.20000000109246940 ) ) ;
#4560=CARTESIAN_POINT ( 'NONE',  ( -1.265664690411616068E-16, 66.06698730000000808, 44.75000000109247367 ) ) ;
#4567=CARTESIAN_POINT ( 'NONE',  ( 2.500000000000002220, 62.96446609406726935, 48.05000000218494449 ) ) ;
#4569=CARTESIAN_POINT ( 'NONE',  ( -0.8561741729129465073, 61.93301270000000613, 45.90000000109247225 ) ) ;
#4585=ORIENTED_EDGE ( 'NONE', *, *, #4915, .F. ) ;
#4587=VECTOR ( 'NONE', #6887, 1000.000000000000000 ) ;
#4594=DIRECTION ( 'NONE',  ( 1.000000000000000000, -0.000000000000000000, 0.000000000000000000 ) ) ;
#4596=CARTESIAN_POINT ( 'NONE',  ( 2.066987300000002303, 63.14382582708705627, 49.10000000109246088 ) ) ;
#4608=VECTOR ( 'NONE', #19314, 1000.000000000000000 ) ;
#4611=CARTESIAN_POINT ( 'NONE',  ( -15.00000000000000000, 47.00000000000000711, 33.99999999999999289 ) ) ;
#4619=ORIENTED_EDGE ( 'NONE', *, *, #13711, .T. ) ;
#4620=ORIENTED_EDGE ( 'NONE', *, *, #7572, .T. ) ;
#4622=VECTOR ( 'NONE', #4019, 1000.000000000000000 ) ;
#4643=VERTEX_POINT ( 'NONE', #12703 ) ;
#4646=CARTESIAN_POINT ( 'NONE',  ( 0.8561741729129460632, 66.06698729999999387, 46.10000000109246798 ) ) ;
#4656=CARTESIAN_POINT ( 'NONE',  ( 0.8561741729129460632, 66.06698730000000808, 47.10000000109246798 ) ) ;
#4658=CARTESIAN_POINT ( 'NONE',  ( 41.00000000000000000, 0.000000000000000000, -50.00000000000000000 ) ) ;
#4669=AXIS2_PLACEMENT_3D ( 'NONE', #17072, #7480, #498 ) ;
#4673=CARTESIAN_POINT ( 'NONE',  ( 0.8561741729129460632, 66.06698729999999387, 46.30000000109247082 ) ) ;
#4684=AXIS2_PLACEMENT_3D ( 'NONE', #16526, #13273, #7506 ) ;
#4686=ORIENTED_EDGE ( 'NONE', *, *, #7810, .F. ) ;
#4687=VERTEX_POINT ( 'NONE', #11414 ) ;
#4689=LINE ( 'NONE', #13591, #4247 ) ;
#4696=VERTEX_POINT ( 'NONE', #15566 ) ;
#4701=ORIENTED_EDGE ( 'NONE', *, *, #15119, .F. ) ;
#4708=EDGE_CURVE ( 'NONE', #17355, #5403, #8390, .T. ) ;
#4715=ORIENTED_EDGE ( 'NONE', *, *, #18463, .F. ) ;
#4723=ORIENTED_EDGE ( 'NONE', *, *, #19188, .T. ) ;
#4729=ORIENTED_EDGE ( 'NONE', *, *, #2528, .F. ) ;
#4730=EDGE_CURVE ( 'NONE', #375, #3539, #19058, .T. ) ;
#4756=LINE ( 'NONE', #10901, #18774 ) ;
#4768=AXIS2_PLACEMENT_3D ( 'NONE', #10193, #1186, #19233 ) ;
#4770=( BOUNDED_SURFACE ( )  B_SPLINE_SURFACE ( 1, 2, ( 
 ( #10453, #3014, #6164, #8990, #18223, #6360, #17821, #14977, #8891, #4596, #18119, #10554, #10650, #4799, #3218, #14881, #9190, #7426, #15178, #16745, #9285, #1655, #13393, #1453, #7730, #1746, #19389, #1840, #3113, #9093, #7629, #15754, #7927, #2226, #5264, #6454, #8115, #1945, #2130, #12612, #8217, #560, #8025, #6550, #14088, #12516, #16844, #11041, #6647, #17039, #841, #3406, #13990, #662, #18517, #12701, #5085, #12323, #14184, #2032, #3596, #9569, #9377, #3693, #15562, #15655, #18319, #18607, #2316, #13890, #5171, #11134, #15371, #749, #3794, #12421, #10944, #18419, #17130, #9664, #6732, #18702, #11220, #17225, #9761, #8299, #466, #14274, #4889, #4985, #10850, #16946, #3510, #9478, #15464, #2792, #15934, #12980, #16221, #8388, #11411 ),
 ( #18788, #16037, #3979, #2697, #2500, #8672, #11702, #8486, #19171, #14362, #937, #8578, #6919, #1224, #8769, #6822, #12890, #5363, #18889, #14654, #14760, #10040, #11605, #2597, #15844, #1036, #7011, #17601, #14557, #4178, #9937, #12790, #11322, #5548, #17317, #3880, #11504, #2406, #17695, #5452, #5645, #17496, #1131, #17407, #13072, #4275, #14464, #4073, #10235, #9846, #18981, #7110, #10130, #19071, #16126, #7206, #13179, #5742, #17903, #16625, #16420, #3191, #6231, #2985, #13667, #8869, #14854, #3084, #1427, #15150, #16720, #1332, #7404, #19270, #13373, #9165, #3290, #4569, #6135, #16521, #10332, #14954, #1528, #12098, #10528, #18094, #4475, #7302, #9260, #58, #10427, #7603, #17996, #13269, #7498, #8967, #1720, #7700, #13474, #6041, #5841 ) ),
 .UNSPECIFIED., .F., .F., .F. ) 
 B_SPLINE_SURFACE_WITH_KNOTS ( ( 2, 2 ),
 ( 3, 2, 2, 2, 2, 2, 2, 2, 2, 2, 2, 2, 2, 2, 2, 2, 2, 2, 2, 2, 2, 2, 2, 2, 2, 2, 2, 2, 2, 2, 2, 2, 2, 2, 2, 2, 2, 2, 2, 2, 2, 2, 2, 2, 2, 2, 2, 2, 2, 2, 3 ),
 ( 0.000000000000000000, 1.000000000000000000 ),
 ( 0.000000000000000000, 0.01785714285714285615, 0.03571428571428571230, 0.05357142857142856845, 0.07142857142857142461, 0.08928571428571428770, 0.1071428571428571369, 0.1250000000000000000, 0.1428571428571428492, 0.1607142857142857262, 0.1785714285714285754, 0.1964285714285714246, 0.2142857142857142738, 0.2321428571428571508, 0.2500000000000000000, 0.2678571428571428492, 0.2857142857142856984, 0.3035714285714285476, 0.3214285714285714524, 0.3392857142857143016, 0.3571428571428571508, 0.3750000000000000000, 0.3928571428571428492, 0.4107142857142856984, 0.4285714285714285476, 0.4464285714285714524, 0.4642857142857143016, 0.4821428571428571508, 0.5000000000000000000, 0.5178571428571429047, 0.5357142857142856984, 0.5535714285714286031, 0.5714285714285713969, 0.5892857142857143016, 0.6071428571428570953, 0.6250000000000000000, 0.6428571428571429047, 0.6607142857142856984, 0.6785714285714286031, 0.6964285714285713969, 0.7142857142857143016, 0.7321428571428570953, 0.7500000000000000000, 0.7678571428571429047, 0.7857142857142856984, 0.8035714285714286031, 0.8214285714285713969, 0.8392857142857143016, 0.8571428571428570953, 0.8750000000000000000, 0.8928571428571429047 ),
 .UNSPECIFIED. ) 
 GEOMETRIC_REPRESENTATION_ITEM ( )  RATIONAL_B_SPLINE_SURFACE ( (
 ( 1.000000000000000000, 0.9238795325112867385, 1.000000000000000000, 0.9238795325112867385, 1.000000000000000000, 0.9238795325112867385, 1.000000000000000000, 0.9238795325112867385, 1.000000000000000000, 0.9238795325112867385, 1.000000000000000000, 0.9238795325112867385, 1.000000000000000000, 0.9238795325112867385, 1.000000000000000000, 0.9238795325112867385, 1.000000000000000000, 0.9238795325112867385, 1.000000000000000000, 0.9238795325112867385, 1.000000000000000000, 0.9238795325112867385, 1.000000000000000000, 0.9238795325112867385, 1.000000000000000000, 0.9238795325112867385, 1.000000000000000000, 0.9238795325112867385, 1.000000000000000000, 0.9238795325112867385, 1.000000000000000000, 0.9238795325112867385, 1.000000000000000000, 0.9238795325112867385, 1.000000000000000000, 0.9238795325112867385, 1.000000000000000000, 0.9238795325112867385, 1.000000000000000000, 0.9238795325112867385, 1.000000000000000000, 0.9238795325112867385, 1.000000000000000000, 0.9238795325112867385, 1.000000000000000000, 0.9238795325112867385, 1.000000000000000000, 0.9238795325112867385, 1.000000000000000000, 0.9238795325112867385, 1.000000000000000000, 0.9238795325112867385, 1.000000000000000000, 0.9238795325112867385, 1.000000000000000000, 0.9238795325112867385, 1.000000000000000000, 0.9238795325112867385, 1.000000000000000000, 0.9238795325112867385, 1.000000000000000000, 0.9238795325112867385, 1.000000000000000000, 0.9238795325112867385, 1.000000000000000000, 0.9238795325112867385, 1.000000000000000000, 0.9238795325112867385, 1.000000000000000000, 0.9238795325112867385, 1.000000000000000000, 0.9238795325112867385, 1.000000000000000000, 0.9238795325112867385, 1.000000000000000000, 0.9238795325112867385, 1.000000000000000000, 0.9238795325112867385, 1.000000000000000000, 0.9238795325112867385, 1.000000000000000000, 0.9238795325112867385, 1.000000000000000000, 0.9238795325112867385, 1.000000000000000000, 0.9238795325112867385, 1.000000000000000000, 0.9238795325112867385, 1.000000000000000000, 0.9238795325112867385, 1.000000000000000000, 0.9238795325112867385, 1.000000000000000000, 0.9238795325112867385, 1.000000000000000000, 0.9238795325112867385, 1.000000000000000000, 0.9238795325112867385, 1.000000000000000000, 0.9238795325112867385, 1.000000000000000000),
 ( 1.000000000000000000, 0.9238795325112867385, 1.000000000000000000, 0.9238795325112867385, 1.000000000000000000, 0.9238795325112867385, 1.000000000000000000, 0.9238795325112867385, 1.000000000000000000, 0.9238795325112867385, 1.000000000000000000, 0.9238795325112867385, 1.000000000000000000, 0.9238795325112867385, 1.000000000000000000, 0.9238795325112867385, 1.000000000000000000, 0.9238795325112867385, 1.000000000000000000, 0.9238795325112867385, 1.000000000000000000, 0.9238795325112867385, 1.000000000000000000, 0.9238795325112867385, 1.000000000000000000, 0.9238795325112867385, 1.000000000000000000, 0.9238795325112867385, 1.000000000000000000, 0.9238795325112867385, 1.000000000000000000, 0.9238795325112867385, 1.000000000000000000, 0.9238795325112867385, 1.000000000000000000, 0.9238795325112867385, 1.000000000000000000, 0.9238795325112867385, 1.000000000000000000, 0.9238795325112867385, 1.000000000000000000, 0.9238795325112867385, 1.000000000000000000, 0.9238795325112867385, 1.000000000000000000, 0.9238795325112867385, 1.000000000000000000, 0.9238795325112867385, 1.000000000000000000, 0.9238795325112867385, 1.000000000000000000, 0.9238795325112867385, 1.000000000000000000, 0.9238795325112867385, 1.000000000000000000, 0.9238795325112867385, 1.000000000000000000, 0.9238795325112867385, 1.000000000000000000, 0.9238795325112867385, 1.000000000000000000, 0.9238795325112867385, 1.000000000000000000, 0.9238795325112867385, 1.000000000000000000, 0.9238795325112867385, 1.000000000000000000, 0.9238795325112867385, 1.000000000000000000, 0.9238795325112867385, 1.000000000000000000, 0.9238795325112867385, 1.000000000000000000, 0.9238795325112867385, 1.000000000000000000, 0.9238795325112867385, 1.000000000000000000, 0.9238795325112867385, 1.000000000000000000, 0.9238795325112867385, 1.000000000000000000, 0.9238795325112867385, 1.000000000000000000, 0.9238795325112867385, 1.000000000000000000, 0.9238795325112867385, 1.000000000000000000, 0.9238795325112867385, 1.000000000000000000, 0.9238795325112867385, 1.000000000000000000, 0.9238795325112867385, 1.000000000000000000, 0.9238795325112867385, 1.000000000000000000, 0.9238795325112867385, 1.000000000000000000, 0.9238795325112867385, 1.000000000000000000, 0.9238795325112867385, 1.000000000000000000) ) ) 
 REPRESENTATION_ITEM ( '' )  SURFACE ( )  );
#4774=CARTESIAN_POINT ( 'NONE',  ( -1.035533905932738863, 61.50000000000000000, 46.25000000218494733 ) ) ;
#4776=CARTESIAN_POINT ( 'NONE',  ( -2.066987300000001415, 64.00000000000000000, 49.75000000109246656 ) ) ;
#4782=CARTESIAN_POINT ( 'NONE',  ( 2.066987300000001415, 64.00000000000000000, 46.95000000109246940 ) ) ;
#4799=CARTESIAN_POINT ( 'NONE',  ( -0.8561741729129465073, 61.93301270000000613, 48.90000000109247225 ) ) ;
#4801=ORIENTED_EDGE ( 'NONE', *, *, #1850, .T. ) ;
#4815=DIRECTION ( 'NONE',  ( 0.000000000000000000, 0.000000000000000000, 1.000000000000000000 ) ) ;
#4816=ORIENTED_EDGE ( 'NONE', *, *, #5923, .F. ) ;
#4820=CARTESIAN_POINT ( 'NONE',  ( -1.461580736456473906, 65.46158073645646880, 49.45000000109246940 ) ) ;
#4828=CARTESIAN_POINT ( 'NONE',  ( 2.499999999999996447, 65.03553390593273775, 46.44999999999999574 ) ) ;
#4829=PLANE ( 'NONE',  #4669 ) ;
#4832=CARTESIAN_POINT ( 'NONE',  ( -32.50000000000000000, 52.00000000000000711, 12.50000000000000000 ) ) ;
#4834=CARTESIAN_POINT ( 'NONE',  ( 2.500000000000001776, 64.00000000000000000, 47.99999999999999289 ) ) ;
#4839=CARTESIAN_POINT ( 'NONE',  ( 32.50000000000000000, 52.00000000000000711, 17.49999999999999645 ) ) ;
#4845=EDGE_LOOP ( 'NONE', ( #5703, #7004 ) ) ;
#4850=EDGE_CURVE ( 'NONE', #232, #13516, #19157, .T. ) ;
#4854=CARTESIAN_POINT ( 'NONE',  ( -32.50000000000000000, 47.00000000000000711, 12.50000000000000000 ) ) ;
#4862=CARTESIAN_POINT ( 'NONE',  ( 4.592425496802577917E-16, 61.50000000000000000, 46.30000000218493739 ) ) ;
#4864=CARTESIAN_POINT ( 'NONE',  ( -2.283493650000001818, 64.00000000000000000, 49.87500000054622973 ) ) ;
#4871=CARTESIAN_POINT ( 'NONE',  ( 1.461580736456473906, 62.53841926354353120, 47.65000000109247225 ) ) ;
#4889=CARTESIAN_POINT ( 'NONE',  ( 2.066987300000001415, 64.00000000000000000, 45.15000000109247225 ) ) ;
#4896=VERTEX_POINT ( 'NONE', #13056 ) ;
#4913=CARTESIAN_POINT ( 'NONE',  ( -2.066987300000001415, 64.00000000000000000, 47.15000000109247225 ) ) ;
#4915=EDGE_CURVE ( 'NONE', #14031, #10014, #8978, .T. ) ;
#4922=DIRECTION ( 'NONE',  ( -0.000000000000000000, 1.000000000000000000, 0.000000000000000000 ) ) ;
#4930=CARTESIAN_POINT ( 'NONE',  ( 1.035533905932738197, 66.50000000000000000, 49.05000000218495160 ) ) ;
#4943=VERTEX_POINT ( 'NONE', #2773 ) ;
#4947=EDGE_CURVE ( 'NONE', #18471, #2469, #2740, .T. ) ;
#4951=CARTESIAN_POINT ( 'NONE',  ( -2.066987300000001415, 64.85617417291294373, 44.90000000109247225 ) ) ;
#4955=DIRECTION ( 'NONE',  ( -0.000000000000000000, 1.000000000000000000, -0.000000000000000000 ) ) ;
#4956=ADVANCED_FACE ( 'NONE', ( #7865 ), #2069, .T. ) ;
#4959=CARTESIAN_POINT ( 'NONE',  ( 1.767766952966370653, 62.23223304703363112, 46.40000000218494591 ) ) ;
#4962=DIRECTION ( 'NONE',  ( -0.8660254037844385966, 0.000000000000000000, 0.5000000000000001110 ) ) ;
#4964=CARTESIAN_POINT ( 'NONE',  ( -24.00000000000000000, 52.00000000000000711, 18.00000000000000000 ) ) ;
#4968=CARTESIAN_POINT ( 'NONE',  ( -1.265664690411616068E-16, 66.06698730000000808, 47.95000000109246940 ) ) ;
#4969=CARTESIAN_POINT ( 'NONE',  ( 2.500000000000001776, 64.00000000000000000, 49.60000000000000142 ) ) ;
#4973=CARTESIAN_POINT ( 'NONE',  ( -32.50000000000000000, 52.00000000000000711, 15.00000000000000000 ) ) ;
#4983=CARTESIAN_POINT ( 'NONE',  ( -15.00000000000000000, 35.00000000000000000, 37.00000000000000000 ) ) ;
#4985=CARTESIAN_POINT ( 'NONE',  ( 2.066987300000002303, 63.14382582708705627, 45.10000000109246798 ) ) ;
#4990=AXIS2_PLACEMENT_3D ( 'NONE', #13555, #10412, #1411 ) ;
#4994=DIRECTION ( 'NONE',  ( -0.000000000000000000, -0.000000000000000000, -1.000000000000000000 ) ) ;
#5001=ORIENTED_EDGE ( 'NONE', *, *, #756, .F. ) ;
#5008=CARTESIAN_POINT ( 'NONE',  ( -0.8561741729129466183, 61.93301270000000613, 48.90000000109247225 ) ) ;
#5010=VERTEX_POINT ( 'NONE', #18260 ) ;
#5025=CARTESIAN_POINT ( 'NONE',  ( 2.500000000000001776, 64.00000000000000000, 49.60000000000000142 ) ) ;
#5030=CARTESIAN_POINT ( 'NONE',  ( 24.00000000000000000, 52.00000000000000711, 18.00000000000000355 ) ) ;
#5050=ADVANCED_FACE ( 'NONE', ( #13924 ), #4829, .T. ) ;
#5055=CARTESIAN_POINT ( 'NONE',  ( 2.500000000000001776, 64.00000000000000000, 45.70000000218494307 ) ) ;
#5063=CARTESIAN_POINT ( 'NONE',  ( 32.50000000000000000, 52.00000000000000711, -32.50000000000000000 ) ) ;
#5065=DIRECTION ( 'NONE',  ( -1.000000000000000000, 0.000000000000000000, 0.000000000000000000 ) ) ;
#5067=CARTESIAN_POINT ( 'NONE',  ( -1.461580736456473906, 65.46158073645646880, 48.05000000109247082 ) ) ;
#5073=CARTESIAN_POINT ( 'NONE',  ( -4.000000000000001776, 67.00000000000000000, 34.99999999999999289 ) ) ;
#5074=ORIENTED_EDGE ( 'NONE', *, *, #5719, .T. ) ;
#5085=CARTESIAN_POINT ( 'NONE',  ( 2.066987300000001415, 64.00000000000000000, 46.75000000109247367 ) ) ;
#5088=ORIENTED_EDGE ( 'NONE', *, *, #1876, .F. ) ;
#5109=DIRECTION ( 'NONE',  ( -0.000000000000000000, -1.000000000000000000, -0.000000000000000000 ) ) ;
#5110=CARTESIAN_POINT ( 'NONE',  ( 0.8561741729129471734, 61.93301270000000613, 48.20000000109247651 ) ) ;
#5114=CARTESIAN_POINT ( 'NONE',  ( -24.00000000000000000, 0.000000000000000000, 18.00000000000000355 ) ) ;
#5148=CARTESIAN_POINT ( 'NONE',  ( -1.767766952966369765, 62.23223304703363112, 45.40000000218494591 ) ) ;
#5151=FACE_OUTER_BOUND ( 'NONE', #2084, .T. ) ;
#5153=LINE ( 'NONE', #5063, #9228 ) ;
#5157=CARTESIAN_POINT ( 'NONE',  ( 2.066987300000001415, 64.00000000000000000, 46.15000000109247225 ) ) ;
#5160=CARTESIAN_POINT ( 'NONE',  ( 32.50000000000000000, 47.00000000000000711, -37.50000000000000711 ) ) ;
#5171=CARTESIAN_POINT ( 'NONE',  ( 1.461580736456473684, 65.46158073645646880, 46.05000000109246372 ) ) ;
#5176=DIRECTION ( 'NONE',  ( 0.000000000000000000, 0.000000000000000000, 1.000000000000000000 ) ) ;
#5186=ORIENTED_EDGE ( 'NONE', *, *, #17646, .F. ) ;
#5225=EDGE_CURVE ( 'NONE', #10014, #3695, #1065, .T. ) ;
#5227=CARTESIAN_POINT ( 'NONE',  ( 2.500000000000001776, 65.03553390593273775, 45.64999999999999147 ) ) ;
#5240=DIRECTION ( 'NONE',  ( 0.000000000000000000, 1.000000000000000000, 0.000000000000000000 ) ) ;
#5242=ADVANCED_FACE ( 'NONE', ( #11640 ), #17631, .T. ) ;
#5245=CARTESIAN_POINT ( 'NONE',  ( 1.461580736456473906, 62.53841926354353120, 47.45000000109246940 ) ) ;
#5250=DIRECTION ( 'NONE',  ( -0.000000000000000000, -0.000000000000000000, -1.000000000000000000 ) ) ;
#5254=CARTESIAN_POINT ( 'NONE',  ( 2.500000000000001776, 64.00000000000000000, 48.79999999999999716 ) ) ;
#5255=CARTESIAN_POINT ( 'NONE',  ( -2.066987300000001415, 64.00000000000000000, 48.95000000109246940 ) ) ;
#5260=CARTESIAN_POINT ( 'NONE',  ( 3.796994071234847710E-16, 61.93301269999999903, 46.55000000109247082 ) ) ;
#5264=CARTESIAN_POINT ( 'NONE',  ( -1.461580736456473906, 65.46158073645646880, 47.85000000109246798 ) ) ;
#5280=ADVANCED_FACE ( 'NONE', ( #18731 ), #13211, .T. ) ;
#5281=EDGE_CURVE ( 'NONE', #10345, #13549, #9972, .T. ) ;
#5289=FACE_OUTER_BOUND ( 'NONE', #8515, .T. ) ;
#5297=CIRCLE ( 'NONE', #4684, 2.499999999999998668 ) ;
#5314=PRESENTATION_STYLE_ASSIGNMENT (( #7062 ) ) ;
#5330=VECTOR ( 'NONE', #4922, 1000.000000000000000 ) ;
#5336=CARTESIAN_POINT ( 'NONE',  ( 2.066987300000002303, 63.14382582708705627, 46.70000000109248361 ) ) ;
#5338=DIRECTION ( 'NONE',  ( 0.000000000000000000, -1.000000000000000000, 0.000000000000000000 ) ) ;
#5345=EDGE_CURVE ( 'NONE', #1624, #964, #14984, .T. ) ;
#5347=CARTESIAN_POINT ( 'NONE',  ( 2.066987300000002303, 63.14382582708705627, 46.10000000109246798 ) ) ;
#5354=B_SPLINE_CURVE_WITH_KNOTS ( 'NONE', 1,
 ( #8727, #1293 ),
 .UNSPECIFIED., .F., .F.,
 ( 2, 2 ),
 ( 0.000000000000000000, 1.000000000000000000 ),
 .UNSPECIFIED. ) ;
#5358=CARTESIAN_POINT ( 'NONE',  ( -2.066987300000001415, 64.00000000000000000, 44.75000000109247367 ) ) ;
#5363=CARTESIAN_POINT ( 'NONE',  ( -2.066987300000001859, 64.85617417291294373, 48.90000000109247225 ) ) ;
#5371=VECTOR ( 'NONE', #8182, 1000.000000000000000 ) ;
#5372=CARTESIAN_POINT ( 'NONE',  ( 4.592425496802577917E-16, 61.50000000000000000, 47.79999999999999716 ) ) ;
#5376=EDGE_LOOP ( 'NONE', ( #3078, #10156, #5705, #14633 ) ) ;
#5381=ORIENTED_EDGE ( 'NONE', *, *, #11287, .T. ) ;
#5401=CARTESIAN_POINT ( 'NONE',  ( -2.500000000000001776, 64.00000000000000000, 46.90000000218494591 ) ) ;
#5403=VERTEX_POINT ( 'NONE', #1558 ) ;
#5409=CARTESIAN_POINT ( 'NONE',  ( -2.500000000000000888, 62.96446609406726935, 45.24999999999999289 ) ) ;
#5416=ORIENTED_EDGE ( 'NONE', *, *, #5451, .T. ) ;
#5419=CARTESIAN_POINT ( 'NONE',  ( 41.00000000000000000, 52.00000000000000711, 18.00000000000000000 ) ) ;
#5428=CARTESIAN_POINT ( 'NONE',  ( -2.066987300000001415, 64.00000000000000000, 48.75000000109246656 ) ) ;
#5441=CARTESIAN_POINT ( 'NONE',  ( -1.461580736456473462, 62.53841926354353120, 45.85000000109246798 ) ) ;
#5442=CARTESIAN_POINT ( 'NONE',  ( -1.461580736456473906, 65.46158073645646880, 48.85000000109246798 ) ) ;
#5447=CARTESIAN_POINT ( 'NONE',  ( -1.265664690411616068E-16, 66.06698730000000808, 45.35000000109246798 ) ) ;
#5451=EDGE_CURVE ( 'NONE', #19196, #14374, #8122, .T. ) ;
#5452=CARTESIAN_POINT ( 'NONE',  ( 2.066987300000001859, 64.85617417291294373, 47.80000000109247082 ) ) ;
#5462=VERTEX_POINT ( 'NONE', #15568 ) ;
#5465=ORIENTED_EDGE ( 'NONE', *, *, #11049, .F. ) ;
#5480=CARTESIAN_POINT ( 'NONE',  ( 0.000000000000000000, 64.00000000000000000, 49.99999999999999289 ) ) ;
#5496=CARTESIAN_POINT ( 'NONE',  ( -2.500000000000001776, 65.03553390593273775, 45.95000000000000995 ) ) ;
#5500=( NAMED_UNIT ( * ) PLANE_ANGLE_UNIT ( ) SI_UNIT ( $, .RADIAN. ) );
#5513=CARTESIAN_POINT ( 'NONE',  ( 2.500000000000001776, 64.00000000000000000, 45.59999999999999432 ) ) ;
#5519=CARTESIAN_POINT ( 'NONE',  ( 3.796994071234847710E-16, 61.93301269999999903, 48.95000000109246940 ) ) ;
#5523=CARTESIAN_POINT ( 'NONE',  ( 32.50000000000000000, 52.00000000000000711, 15.00000000000000000 ) ) ;
#5534=CARTESIAN_POINT ( 'NONE',  ( 2.066987300000002303, 63.14382582708705627, 45.30000000109247082 ) ) ;
#5535=CARTESIAN_POINT ( 'NONE',  ( 2.066987300000001415, 64.85617417291294373, 48.60000000109246798 ) ) ;
#5544=CARTESIAN_POINT ( 'NONE',  ( -0.8561741729129461742, 66.06698730000000808, 44.60000000109246798 ) ) ;
#5548=CARTESIAN_POINT ( 'NONE',  ( -2.066987300000001859, 64.85617417291294373, 48.10000000109246798 ) ) ;
#5551=CARTESIAN_POINT ( 'NONE',  ( 1.767766952966370653, 62.23223304703363112, 45.60000000218494165 ) ) ;
#5553=CARTESIAN_POINT ( 'NONE',  ( 2.500000000000001776, 64.00000000000000000, 49.99999999999999289 ) ) ;
#5561=( NAMED_UNIT ( * ) SI_UNIT ( $, .STERADIAN. ) SOLID_ANGLE_UNIT ( ) );
#5566=EDGE_CURVE ( 'NONE', #13223, #2714, #5297, .T. ) ;
#5584=ORIENTED_EDGE ( 'NONE', *, *, #4850, .T. ) ;
#5598=CARTESIAN_POINT ( 'NONE',  ( 2.500000000000001776, 64.00000000000000000, 46.50000000218494733 ) ) ;
#5603=CARTESIAN_POINT ( 'NONE',  ( 2.500000000000010658, 62.96446609406726225, 48.05000000218495160 ) ) ;
#5606=CARTESIAN_POINT ( 'NONE',  ( -1.530808498934192803E-16, 66.50000000000000000, 48.30000000218494449 ) ) ;
#5612=FACE_OUTER_BOUND ( 'NONE', #2124, .T. ) ;
#5617=VECTOR ( 'NONE', #7961, 1000.000000000000000 ) ;
#5618=CARTESIAN_POINT ( 'NONE',  ( 0.8561741729129460632, 66.06698729999999387, 46.90000000109247225 ) ) ;
#5629=CARTESIAN_POINT ( 'NONE',  ( 2.500000000000001776, 64.00000000000000000, 47.99999999999999289 ) ) ;
#5630=CARTESIAN_POINT ( 'NONE',  ( 0.8561741729129460632, 66.06698730000000808, 49.50000000109246656 ) ) ;
#5645=CARTESIAN_POINT ( 'NONE',  ( 2.066987300000001415, 64.00000000000000000, 47.75000000109246656 ) ) ;
#5647=CARTESIAN_POINT ( 'NONE',  ( -1.035533905932738863, 61.50000000000000000, 45.45000000218494307 ) ) ;
#5648=COLOUR_RGB ( '', 0.66274510, 0.83137255, 0.94901961) ;
#5663=ORIENTED_EDGE ( 'NONE', *, *, #165, .T. ) ;
#5676=EDGE_LOOP ( 'NONE', ( #13004, #12939, #11992, #12629 ) ) ;
#5691=AXIS2_PLACEMENT_3D ( 'NONE', #11192, #902, #11290 ) ;
#5692=CARTESIAN_POINT ( 'NONE',  ( -1.530808498934192803E-16, 66.50000000000000000, 45.00000000000000000 ) ) ;
#5696=CARTESIAN_POINT ( 'NONE',  ( -2.500000000000006661, 65.03553390593272354, 45.14999999999999858 ) ) ;
#5699=ADVANCED_FACE ( 'NONE', ( #13184 ), #8863, .T. ) ;
#5703=ORIENTED_EDGE ( 'NONE', *, *, #851, .F. ) ;
#5705=ORIENTED_EDGE ( 'NONE', *, *, #6177, .T. ) ;
#5708=VECTOR ( 'NONE', #18099, 1000.000000000000000 ) ;
#5711=FACE_OUTER_BOUND ( 'NONE', #8079, .T. ) ;
#5719=EDGE_CURVE ( 'NONE', #1836, #9208, #9805, .T. ) ;
#5720=CARTESIAN_POINT ( 'NONE',  ( 1.461580736456473906, 62.53841926354353120, 45.05000000109246372 ) ) ;
#5724=FACE_BOUND ( 'NONE', #1216, .T. ) ;
#5731=CARTESIAN_POINT ( 'NONE',  ( 4.592425496802577917E-16, 61.50000000000000000, 46.19999999999999574 ) ) ;
#5732=CARTESIAN_POINT ( 'NONE',  ( -0.8561741729129466183, 61.93301270000000613, 48.30000000109247082 ) ) ;
#5742=CARTESIAN_POINT ( 'NONE',  ( 2.066987300000002303, 63.14382582708705627, 46.90000000109247225 ) ) ;
#5748=CARTESIAN_POINT ( 'NONE',  ( 0.000000000000000000, 0.000000000000000000, 34.99999999999999289 ) ) ;
#5751=CARTESIAN_POINT ( 'NONE',  ( -2.500000000000001776, 64.00000000000000000, 44.50000000218494733 ) ) ;
#5769=EDGE_LOOP ( 'NONE', ( #15070, #2435, #5913, #1763 ) ) ;
#5771=CARTESIAN_POINT ( 'NONE',  ( -1.464522546803548496E-16, 66.39174682499999847, 44.93750000027311842 ) ) ;
#5777=CARTESIAN_POINT ( 'NONE',  ( 2.500000000000001776, 64.00000000000000000, 49.99999999999999289 ) ) ;
#5791=ORIENTED_EDGE ( 'NONE', *, *, #8655, .F. ) ;
#5805=DIRECTION ( 'NONE',  ( 0.000000000000000000, 0.000000000000000000, -1.000000000000000000 ) ) ;
#5812=AXIS2_PLACEMENT_3D ( 'NONE', #10451, #1743, #16350 ) ;
#5817=ORIENTED_EDGE ( 'NONE', *, *, #9803, .F. ) ;
#5823=FACE_BOUND ( 'NONE', #12544, .T. ) ;
#5825=CARTESIAN_POINT ( 'NONE',  ( 1.035533905932739751, 61.50000000000000000, 47.04999999999999005 ) ) ;
#5826=CARTESIAN_POINT ( 'NONE',  ( -1.461580736456473462, 62.53841926354353120, 46.65000000109247225 ) ) ;
#5828=VECTOR ( 'NONE', #4955, 1000.000000000000000 ) ;
#5837=CARTESIAN_POINT ( 'NONE',  ( 1.035533905932739751, 61.50000000000000000, 48.75000000218494023 ) ) ;
#5839=AXIS2_PLACEMENT_3D ( 'NONE', #11972, #10595, #8733 ) ;
#5841=CARTESIAN_POINT ( 'NONE',  ( -1.265664690411616068E-16, 66.06698730000000808, 44.75000000109247367 ) ) ;
#5849=CARTESIAN_POINT ( 'NONE',  ( -24.00000000000000000, 47.00000000000000711, 18.00000000000000355 ) ) ;
#5859=ORIENTED_EDGE ( 'NONE', *, *, #1853, .F. ) ;
#5868=CARTESIAN_POINT ( 'NONE',  ( -1.767766952966369765, 62.23223304703363112, 46.89999999999999858 ) ) ;
#5877=EDGE_LOOP ( 'NONE', ( #14602, #15858, #10852, #7263, #3734 ) ) ;
#5889=ORIENTED_EDGE ( 'NONE', *, *, #16114, .F. ) ;
#5892=CARTESIAN_POINT ( 'NONE',  ( -2.500000000000011546, 65.03553390593272354, 44.45000000218495018 ) ) ;
#5902=CARTESIAN_POINT ( 'NONE',  ( 1.035533905932738197, 66.50000000000000000, 48.14999999999999858 ) ) ;
#5911=AXIS2_PLACEMENT_3D ( 'NONE', #3580, #251, #5065 ) ;
#5913=ORIENTED_EDGE ( 'NONE', *, *, #5281, .T. ) ;
#5922=CARTESIAN_POINT ( 'NONE',  ( -0.8561741729129466183, 61.93301270000000613, 45.90000000109247225 ) ) ;
#5923=EDGE_CURVE ( 'NONE', #8404, #4643, #18049, .T. ) ;
#5962=AXIS2_PLACEMENT_3D ( 'NONE', #5523, #11042, #6551 ) ;
#5963=CARTESIAN_POINT ( 'NONE',  ( -1.265664690411616068E-16, 66.06698730000000808, 44.75000000109247367 ) ) ;
#5974=AXIS2_PLACEMENT_3D ( 'NONE', #19307, #17834, #13513 ) ;
#5979=ORIENTED_EDGE ( 'NONE', *, *, #15135, .F. ) ;
#5988=AXIS2_PLACEMENT_3D ( 'NONE', #14865, #13382, #11919 ) ;
#5996=ORIENTED_EDGE ( 'NONE', *, *, #9440, .F. ) ;
#6007=CARTESIAN_POINT ( 'NONE',  ( -2.500000000000001776, 65.03553390593273775, 49.94999999999998863 ) ) ;
#6020=ORIENTED_EDGE ( 'NONE', *, *, #387, .F. ) ;
#6023=PLANE ( 'NONE',  #10295 ) ;
#6028=CARTESIAN_POINT ( 'NONE',  ( 2.066987300000001415, 64.85617417291294373, 45.40000000109247225 ) ) ;
#6035=EDGE_CURVE ( 'NONE', #2469, #19221, #1495, .T. ) ;
#6038=CARTESIAN_POINT ( 'NONE',  ( 2.500000000000002220, 62.96446609406726935, 48.85000000218494165 ) ) ;
#6041=CARTESIAN_POINT ( 'NONE',  ( -0.8561741729129461742, 66.06698729999999387, 44.80000000109246372 ) ) ;
#6050=DIRECTION ( 'NONE',  ( -0.000000000000000000, 0.000000000000000000, 1.000000000000000000 ) ) ;
#6052=ORIENTED_EDGE ( 'NONE', *, *, #1617, .T. ) ;
#6071=DIRECTION ( 'NONE',  ( 0.000000000000000000, 1.000000000000000000, 0.000000000000000000 ) ) ;
#6076=EDGE_CURVE ( 'NONE', #14374, #4696, #7617, .T. ) ;
#6097=CARTESIAN_POINT ( 'NONE',  ( -15.00000000000000000, 47.00000000000000711, 33.99999999999999289 ) ) ;
#6109=CARTESIAN_POINT ( 'NONE',  ( -0.8561741729129465073, 61.93301270000000613, 44.90000000109247225 ) ) ;
#6120=CARTESIAN_POINT ( 'NONE',  ( 1.461580736456473906, 62.53841926354353120, 47.65000000109247225 ) ) ;
#6127=EDGE_CURVE ( 'NONE', #17145, #3695, #13755, .T. ) ;
#6132=CARTESIAN_POINT ( 'NONE',  ( -2.500000000000000888, 62.96446609406726935, 48.55000000218494449 ) ) ;
#6135=CARTESIAN_POINT ( 'NONE',  ( -1.461580736456473462, 62.53841926354353120, 45.85000000109246798 ) ) ;
#6144=CARTESIAN_POINT ( 'NONE',  ( 2.066987300000001859, 64.85617417291294373, 47.80000000109247082 ) ) ;
#6162=CARTESIAN_POINT ( 'NONE',  ( -1.265664690411616068E-16, 66.06698730000000808, 44.75000000109247367 ) ) ;
#6164=CARTESIAN_POINT ( 'NONE',  ( -1.461580736456473906, 65.46158073645646880, 49.45000000109246940 ) ) ;
#6169=ORIENTED_EDGE ( 'NONE', *, *, #13265, .T. ) ;
#6177=EDGE_CURVE ( 'NONE', #6482, #8924, #16108, .T. ) ;
#6191=CARTESIAN_POINT ( 'NONE',  ( -1.461580736456473906, 65.46158073645646880, 47.85000000109246798 ) ) ;
#6192=CARTESIAN_POINT ( 'NONE',  ( -41.00000000000000000, 0.000000000000000000, -67.72004514666936359 ) ) ;
#6209=ORIENTED_EDGE ( 'NONE', *, *, #17847, .F. ) ;
#6211=CARTESIAN_POINT ( 'NONE',  ( -1.530808498934192803E-16, 66.50000000000000000, 47.39999999999999858 ) ) ;
#6217=ADVANCED_FACE ( 'NONE', ( #16403 ), #9048, .T. ) ;
#6221=CARTESIAN_POINT ( 'NONE',  ( 1.461580736456473906, 62.53841926354353120, 45.25000000109247367 ) ) ;
#6226=VECTOR ( 'NONE', #8102, 1000.000000000000000 ) ;
#6229=CARTESIAN_POINT ( 'NONE',  ( -1.530808498934192803E-16, 66.50000000000000000, 44.30000000218494449 ) ) ;
#6231=CARTESIAN_POINT ( 'NONE',  ( -1.461580736456473462, 62.53841926354353120, 46.65000000109247225 ) ) ;
#6238=CARTESIAN_POINT ( 'NONE',  ( -1.461580736456473906, 65.46158073645646880, 47.25000000109246656 ) ) ;
#6255=VECTOR ( 'NONE', #3656, 1000.000000000000000 ) ;
#6260=VERTEX_POINT ( 'NONE', #2968 ) ;
#6261=CYLINDRICAL_SURFACE ( 'NONE', #932, 2.999999999999999112 ) ;
#6266=ADVANCED_FACE ( 'NONE', ( #12081 ), #6023, .F. ) ;
#6282=CARTESIAN_POINT ( 'NONE',  ( 1.461580736456473906, 62.53841926354353120, 48.25000000109246656 ) ) ;
#6284=ORIENTED_EDGE ( 'NONE', *, *, #10219, .F. ) ;
#6287=VECTOR ( 'NONE', #16164, 1000.000000000000000 ) ;
#6293=CARTESIAN_POINT ( 'NONE',  ( 1.035533905932738197, 66.50000000000000000, 46.54999999999999716 ) ) ;
#6313=ORIENTED_EDGE ( 'NONE', *, *, #6867, .T. ) ;
#6318=CARTESIAN_POINT ( 'NONE',  ( -4.000000000000001776, 67.00000000000000000, 30.00000000000000000 ) ) ;
#6329=EDGE_LOOP ( 'NONE', ( #5416, #8401, #15992, #11647, #12021, #4585, #6020, #15429, #9022, #333, #1546, #10261, #792, #3128, #7036, #10853 ) ) ;
#6333=CARTESIAN_POINT ( 'NONE',  ( 1.035533905932739751, 61.50000000000000000, 44.75000000218494023 ) ) ;
#6341=CYLINDRICAL_SURFACE ( 'NONE', #7899, 2.500000000000001776 ) ;
#6342=CARTESIAN_POINT ( 'NONE',  ( -2.066987300000001415, 64.00000000000000000, 48.15000000109247225 ) ) ;
#6360=CARTESIAN_POINT ( 'NONE',  ( 0.8561741729129460632, 66.06698729999999387, 49.30000000109246372 ) ) ;
#6362=ORIENTED_EDGE ( 'NONE', *, *, #9870, .T. ) ;
#6364=FACE_OUTER_BOUND ( 'NONE', #4387, .T. ) ;
#6376=VERTEX_POINT ( 'NONE', #6610 ) ;
#6382=CARTESIAN_POINT ( 'NONE',  ( -1.461580736456473462, 62.53841926354353120, 47.25000000109247367 ) ) ;
#6383=CARTESIAN_POINT ( 'NONE',  ( 14.99999999999998579, 73.00000000000001421, 23.99999999999997158 ) ) ;
#6404=LINE ( 'NONE', #9521, #6783 ) ;
#6417=CARTESIAN_POINT ( 'NONE',  ( -2.066987300000000971, 63.14382582708704916, 45.00000000109247367 ) ) ;
#6427=CARTESIAN_POINT ( 'NONE',  ( 2.500000000000002220, 62.96446609406726935, 46.45000000218495018 ) ) ;
#6429=DIRECTION ( 'NONE',  ( -1.000000000000000000, 0.000000000000000000, 0.000000000000000000 ) ) ;
#6436=CARTESIAN_POINT ( 'NONE',  ( 2.066987300000002303, 63.14382582708705627, 48.50000000109246656 ) ) ;
#6440=CARTESIAN_POINT ( 'NONE',  ( -14.99999999999999645, 73.00000000000001421, 23.99999999999997868 ) ) ;
#6450=LINE ( 'NONE', #6547, #16462 ) ;
#6454=CARTESIAN_POINT ( 'NONE',  ( -0.8561741729129461742, 66.06698729999999387, 47.80000000109247082 ) ) ;
#6465=VECTOR ( 'NONE', #5240, 1000.000000000000000 ) ;
#6476=CARTESIAN_POINT ( 'NONE',  ( -1.461580736456473462, 62.53841926354353120, 48.05000000109247082 ) ) ;
#6477=LINE ( 'NONE', #8141, #14716 ) ;
#6482=VERTEX_POINT ( 'NONE', #11467 ) ;
#6492=CARTESIAN_POINT ( 'NONE',  ( -1.035533905932738641, 66.50000000000000000, 49.15000000218494591 ) ) ;
#6493=CARTESIAN_POINT ( 'NONE',  ( 14.99999999999998579, 47.00000000000000711, 20.99999999999997513 ) ) ;
#6495=CARTESIAN_POINT ( 'NONE',  ( -1.530808498934192803E-16, 66.50000000000000000, 49.79999999999999716 ) ) ;
#6501=CARTESIAN_POINT ( 'NONE',  ( -32.50000000000000000, 47.00000000000000711, -37.50000000000000711 ) ) ;
#6511=CARTESIAN_POINT ( 'NONE',  ( -2.500000000000001776, 64.00000000000000000, 46.00000000000000000 ) ) ;
#6520=CARTESIAN_POINT ( 'NONE',  ( 2.500000000000001776, 65.03553390593273775, 46.55000000218494449 ) ) ;
#6531=CARTESIAN_POINT ( 'NONE',  ( 0.8561741729129472844, 61.93301270000000613, 47.60000000109246798 ) ) ;
#6537=CYLINDRICAL_SURFACE ( 'NONE', #11122, 2.499999999999998668 ) ;
#6547=CARTESIAN_POINT ( 'NONE',  ( -32.50000000000000000, 52.00000000000000711, 17.49999999999999645 ) ) ;
#6550=CARTESIAN_POINT ( 'NONE',  ( 0.8561741729129472844, 61.93301270000000613, 47.40000000109247225 ) ) ;
#6551=DIRECTION ( 'NONE',  ( 0.000000000000000000, 0.000000000000000000, 1.000000000000000000 ) ) ;
#6574=LINE ( 'NONE', #3623, #14156 ) ;
#6575=CARTESIAN_POINT ( 'NONE',  ( 2.066987300000001415, 64.00000000000000000, 48.35000000109246798 ) ) ;
#6584=DIRECTION ( 'NONE',  ( -0.000000000000000000, 1.000000000000000000, -0.000000000000000000 ) ) ;
#6593=CIRCLE ( 'NONE', #12523, 2.500000000000002220 ) ;
#6610=CARTESIAN_POINT ( 'NONE',  ( -2.500000000000001776, 64.00000000000000000, 48.50000000218494023 ) ) ;
#6621=CARTESIAN_POINT ( 'NONE',  ( 1.035533905932738197, 66.50000000000000000, 46.65000000218494591 ) ) ;
#6632=CARTESIAN_POINT ( 'NONE',  ( 2.066987300000001415, 64.00000000000000000, 45.35000000109246798 ) ) ;
#6634=DIRECTION ( 'NONE',  ( 1.000000000000000000, 0.000000000000000000, 0.000000000000000000 ) ) ;
#6647=CARTESIAN_POINT ( 'NONE',  ( -2.066987300000001415, 64.00000000000000000, 47.15000000109247225 ) ) ;
#6652=CARTESIAN_POINT ( 'NONE',  ( 4.000000000000003553, 47.00000000000000711, 34.99999999999999289 ) ) ;
#6654=CYLINDRICAL_SURFACE ( 'NONE', #12806, 2.500000000000001776 ) ;
#6664=ORIENTED_EDGE ( 'NONE', *, *, #1001, .F. ) ;
#6687=ORIENTED_EDGE ( 'NONE', *, *, #12110, .F. ) ;
#6690=ORIENTED_EDGE ( 'NONE', *, *, #9803, .T. ) ;
#6692=CARTESIAN_POINT ( 'NONE',  ( 4.592425496802577917E-16, 61.50000000000000000, 45.39999999999999858 ) ) ;
#6695=CYLINDRICAL_SURFACE ( 'NONE', #15978, 2.999999999999999112 ) ;
#6700=CARTESIAN_POINT ( 'NONE',  ( 1.767766952966369987, 65.76776695296638309, 45.80000000218493739 ) ) ;
#6703=CARTESIAN_POINT ( 'NONE',  ( 41.00000000000000000, 47.00000000000000711, 30.00000000000000000 ) ) ;
#6706=EDGE_CURVE ( 'NONE', #16534, #2938, #1587, .T. ) ;
#6707=CARTESIAN_POINT ( 'NONE',  ( -1.265664690411616068E-16, 66.06698730000000808, 48.55000000109247082 ) ) ;
#6710=CARTESIAN_POINT ( 'NONE',  ( 0.000000000000000000, 64.00000000000000000, 49.99999999999999289 ) ) ;
#6712=DIRECTION ( 'NONE',  ( -1.000000000000000000, 0.000000000000000000, 0.000000000000000000 ) ) ;
#6716=CARTESIAN_POINT ( 'NONE',  ( 0.8561741729129472844, 61.93301270000000613, 45.20000000109248361 ) ) ;
#6718=PLANE ( 'NONE',  #4768 ) ;
#6725=EDGE_CURVE ( 'NONE', #16897, #13230, #3153, .T. ) ;
#6727=CARTESIAN_POINT ( 'NONE',  ( 2.066987300000001415, 64.00000000000000000, 46.75000000109247367 ) ) ;
#6732=CARTESIAN_POINT ( 'NONE',  ( -2.066987300000001415, 64.00000000000000000, 45.55000000109246372 ) ) ;
#6737=DIRECTION ( 'NONE',  ( -0.000000000000000000, -0.000000000000000000, -1.000000000000000000 ) ) ;
#6754=( BOUNDED_CURVE ( )  B_SPLINE_CURVE ( 2, ( #9740, #11585, #18869, #2477, #17383, #6805, #1107, #3956, #13052 ),
 .UNSPECIFIED., .F., .F. ) 
 B_SPLINE_CURVE_WITH_KNOTS ( ( 3, 2, 2, 2, 3 ),
 ( 0.4999999999999999445, 0.5178571428571427937, 0.5357142857142855874, 0.5535714285714283811, 0.5714285714285711748 ),
 .UNSPECIFIED. ) 
 CURVE ( )  GEOMETRIC_REPRESENTATION_ITEM ( )  RATIONAL_B_SPLINE_CURVE ( ( 1.000000000000000222, 0.9238795325112865164, 1.000000000000000000, 0.9238795325112867385, 1.000000000000000000, 0.9238795325112867385, 1.000000000000000000, 0.9238795325112877377, 0.9999999999999990008 ) ) 
 REPRESENTATION_ITEM ( '' )  );
#6767=DIRECTION ( 'NONE',  ( -1.000000000000000000, 0.000000000000000000, 0.000000000000000000 ) ) ;
#6768=LINE ( 'NONE', #6852, #5617 ) ;
#6774=CARTESIAN_POINT ( 'NONE',  ( 2.500000000000001776, 64.00000000000000000, 49.99999999999999289 ) ) ;
#6783=VECTOR ( 'NONE', #15510, 1000.000000000000000 ) ;
#6786=EDGE_CURVE ( 'NONE', #13006, #17737, #12128, .T. ) ;
#6803=CARTESIAN_POINT ( 'NONE',  ( -1.461580736456473462, 62.53841926354353120, 46.45000000109246940 ) ) ;
#6805=CARTESIAN_POINT ( 'NONE',  ( -1.035533905932738863, 61.50000000000000000, 46.25000000218494733 ) ) ;
#6811=CARTESIAN_POINT ( 'NONE',  ( 4.592425496802577917E-16, 61.50000000000000000, 49.39999999999999147 ) ) ;
#6815=CARTESIAN_POINT ( 'NONE',  ( -10.00000000000000000, 47.00000000000000711, 33.99999999999999289 ) ) ;
#6818=CARTESIAN_POINT ( 'NONE',  ( 0.8561741729129471734, 61.93301270000000613, 45.80000000109246372 ) ) ;
#6822=CARTESIAN_POINT ( 'NONE',  ( -2.066987300000001415, 63.14382582708705627, 49.00000000109246656 ) ) ;
#6832=ORIENTED_EDGE ( 'NONE', *, *, #7881, .F. ) ;
#6840=VECTOR ( 'NONE', #2207, 1000.000000000000000 ) ;
#6844=EDGE_LOOP ( 'NONE', ( #14973, #18165, #12468, #16963 ) ) ;
#6852=CARTESIAN_POINT ( 'NONE',  ( -24.00000000000000000, 47.00000000000000711, -67.72004514666936359 ) ) ;
#6867=EDGE_CURVE ( 'NONE', #17639, #3710, #307, .T. ) ;
#6868=AXIS2_PLACEMENT_3D ( 'NONE', #14837, #131, #1511 ) ;
#6872=AXIS2_PLACEMENT_3D ( 'NONE', #7583, #12079, #1313 ) ;
#6873=CARTESIAN_POINT ( 'NONE',  ( -2.500000000000001776, 64.00000000000000000, 49.19999999999999574 ) ) ;
#6879=LINE ( 'NONE', #5419, #9111 ) ;
#6887=DIRECTION ( 'NONE',  ( -2.602085213965211135E-16, 1.000000000000000000, -0.000000000000000000 ) ) ;
#6889=ORIENTED_EDGE ( 'NONE', *, *, #8671, .F. ) ;
#6893=CARTESIAN_POINT ( 'NONE',  ( 0.8561741729129460632, 66.06698729999999387, 48.50000000109246656 ) ) ;
#6896=AXIS2_PLACEMENT_3D ( 'NONE', #10488, #2852, #11856 ) ;
#6904=CARTESIAN_POINT ( 'NONE',  ( -1.265664690411616068E-16, 66.06698730000000808, 45.55000000109246372 ) ) ;
#6908=LINE ( 'NONE', #8568, #4286 ) ;
#6910=LINE ( 'NONE', #15744, #12689 ) ;
#6913=CARTESIAN_POINT ( 'NONE',  ( 0.000000000000000000, 64.00000000000000000, 34.99999999999999289 ) ) ;
#6919=CARTESIAN_POINT ( 'NONE',  ( 3.796994071234847710E-16, 61.93301269999999903, 49.15000000109246514 ) ) ;
#6929=DIRECTION ( 'NONE',  ( 1.000000000000000000, 0.000000000000000000, 0.000000000000000000 ) ) ;
#6971=CARTESIAN_POINT ( 'NONE',  ( -1.767766952966370209, 65.76776695296638309, 46.80000000218494449 ) ) ;
#6976=ADVANCED_FACE ( 'NONE', ( #1348 ), #16237, .T. ) ;
#6987=CARTESIAN_POINT ( 'NONE',  ( -1.461580736456473906, 65.46158073645646880, 48.65000000109247225 ) ) ;
#6999=CARTESIAN_POINT ( 'NONE',  ( -1.530808498934192803E-16, 66.50000000000000000, 49.79999999999999716 ) ) ;
#7000=CARTESIAN_POINT ( 'NONE',  ( -41.00000000000000000, 52.00000000000000711, -50.00000000000000000 ) ) ;
#7001=ADVANCED_FACE ( 'NONE', ( #13493 ), #1649, .T. ) ;
#7004=ORIENTED_EDGE ( 'NONE', *, *, #165, .F. ) ;
#7006=CARTESIAN_POINT ( 'NONE',  ( -1.461580736456473462, 62.53841926354353120, 44.85000000109246798 ) ) ;
#7011=CARTESIAN_POINT ( 'NONE',  ( 1.461580736456473906, 62.53841926354353120, 48.45000000109246940 ) ) ;
#7025=( NAMED_UNIT ( * ) PLANE_ANGLE_UNIT ( ) SI_UNIT ( $, .RADIAN. ) );
#7027=VERTEX_POINT ( 'NONE', #11625 ) ;
#7036=ORIENTED_EDGE ( 'NONE', *, *, #16592, .F. ) ;
#7047=CARTESIAN_POINT ( 'NONE',  ( 2.500000000000001776, 64.00000000000000000, 47.30000000218494449 ) ) ;
#7054=LINE ( 'NONE', #2361, #16819 ) ;
#7057=CARTESIAN_POINT ( 'NONE',  ( -1.767766952966369765, 62.23223304703363112, 45.29999999999999005 ) ) ;
#7062=SURFACE_STYLE_USAGE ( .BOTH. , #2646 ) ;
#7071=CARTESIAN_POINT ( 'NONE',  ( -1.035533905932738641, 66.50000000000000000, 48.35000000218494165 ) ) ;
#7077=AXIS2_PLACEMENT_3D ( 'NONE', #2862, #8841, #19339 ) ;
#7083=CARTESIAN_POINT ( 'NONE',  ( 2.066987300000001415, 64.00000000000000000, 47.55000000109247082 ) ) ;
#7091=VECTOR ( 'NONE', #16372, 1000.000000000000000 ) ;
#7096=CARTESIAN_POINT ( 'NONE',  ( 1.767766952966370653, 62.23223304703363112, 47.89999999999999858 ) ) ;
#7097=CARTESIAN_POINT ( 'NONE',  ( 2.066987300000001415, 64.00000000000000000, 49.35000000109246798 ) ) ;
#7101=VERTEX_POINT ( 'NONE', #11395 ) ;
#7110=CARTESIAN_POINT ( 'NONE',  ( -0.8561741729129461742, 66.06698729999999387, 47.20000000109247651 ) ) ;
#7113=CARTESIAN_POINT ( 'NONE',  ( -14.99999999999999645, 47.00000000000000711, 26.99999999999997868 ) ) ;
#7121=ORIENTED_EDGE ( 'NONE', *, *, #3967, .F. ) ;
#7125=EDGE_LOOP ( 'NONE', ( #9588, #17744, #13529, #3241 ) ) ;
#7132=FACE_OUTER_BOUND ( 'NONE', #1988, .T. ) ;
#7154=CARTESIAN_POINT ( 'NONE',  ( -1.035533905932738641, 66.50000000000000000, 45.04999999999999005 ) ) ;
#7158=CARTESIAN_POINT ( 'NONE',  ( -15.00000000000000000, 0.000000000000000000, 0.000000000000000000 ) ) ;
#7160=LINE ( 'NONE', #7455, #12201 ) ;
#7189=CARTESIAN_POINT ( 'NONE',  ( 1.767766952966369987, 65.76776695296638309, 48.09999999999999432 ) ) ;
#7203=CARTESIAN_POINT ( 'NONE',  ( 3.999999999999998224, 67.00000000000000000, 34.99999999999999289 ) ) ;
#7206=CARTESIAN_POINT ( 'NONE',  ( 2.066987300000001859, 64.85617417291294373, 47.00000000109246656 ) ) ;
#7220=CARTESIAN_POINT ( 'NONE',  ( -1.767766952966369765, 62.23223304703363112, 44.60000000218494165 ) ) ;
#7228=EDGE_LOOP ( 'NONE', ( #10844, #419, #8313, #5817 ) ) ;
#7231=VECTOR ( 'NONE', #3940, 1000.000000000000000 ) ;
#7237=ORIENTED_EDGE ( 'NONE', *, *, #5345, .F. ) ;
#7240=DIRECTION ( 'NONE',  ( 1.000000000000000000, 0.000000000000000000, 0.000000000000000000 ) ) ;
#7248=CARTESIAN_POINT ( 'NONE',  ( -2.499999999999996003, 62.96446609406726225, 46.95000000218494307 ) ) ;
#7251=ORIENTED_EDGE ( 'NONE', *, *, #7610, .T. ) ;
#7262=CARTESIAN_POINT ( 'NONE',  ( 1.767766952966369987, 65.76776695296638309, 47.40000000218494591 ) ) ;
#7263=ORIENTED_EDGE ( 'NONE', *, *, #7572, .F. ) ;
#7265=ORIENTED_EDGE ( 'NONE', *, *, #14625, .T. ) ;
#7277=DIRECTION ( 'NONE',  ( 0.000000000000000000, 1.000000000000000000, -0.000000000000000000 ) ) ;
#7281=CARTESIAN_POINT ( 'NONE',  ( -0.8561741729129461742, 66.06698729999999387, 45.40000000109246514 ) ) ;
#7290=FACE_BOUND ( 'NONE', #14670, .T. ) ;
#7292=CARTESIAN_POINT ( 'NONE',  ( -1.035533905932738641, 66.50000000000000000, 47.44999999999999574 ) ) ;
#7293=CARTESIAN_POINT ( 'NONE',  ( 3.796994071234847710E-16, 61.93301269999999903, 47.55000000109247082 ) ) ;
#7300=CARTESIAN_POINT ( 'NONE',  ( 1.767766952966370653, 62.23223304703363112, 48.00000000218494023 ) ) ;
#7302=CARTESIAN_POINT ( 'NONE',  ( 2.066987300000001859, 64.85617417291294373, 45.40000000109246514 ) ) ;
#7313=ADVANCED_FACE ( 'NONE', ( #3275 ), #17096, .T. ) ;
#7314=CARTESIAN_POINT ( 'NONE',  ( -1.035533905932738863, 61.50000000000000000, 44.65000000218493881 ) ) ;
#7322=EDGE_LOOP ( 'NONE', ( #3933, #1455, #18135, #10308, #9181 ) ) ;
#7362=ORIENTED_EDGE ( 'NONE', *, *, #5451, .F. ) ;
#7371=ORIENTED_EDGE ( 'NONE', *, *, #6706, .F. ) ;
#7378=CARTESIAN_POINT ( 'NONE',  ( -1.461580736456473906, 65.46158073645646880, 46.25000000109247367 ) ) ;
#7386=CARTESIAN_POINT ( 'NONE',  ( 1.767766952966369987, 65.76776695296638309, 45.00000000218494733 ) ) ;
#7388=CARTESIAN_POINT ( 'NONE',  ( 2.500000000000001776, 64.00000000000000000, 46.39999999999999858 ) ) ;
#7389=CARTESIAN_POINT ( 'NONE',  ( 2.066987300000001859, 63.14382582708704916, 46.90000000109247225 ) ) ;
#7403=AXIS2_PLACEMENT_3D ( 'NONE', #13840, #17169, #12740 ) ;
#7404=CARTESIAN_POINT ( 'NONE',  ( 2.066987300000001415, 64.00000000000000000, 46.15000000109247225 ) ) ;
#7418=ORIENTED_EDGE ( 'NONE', *, *, #8414, .T. ) ;
#7426=CARTESIAN_POINT ( 'NONE',  ( -2.066987300000001859, 64.85617417291294373, 48.70000000109247651 ) ) ;
#7438=EDGE_CURVE ( 'NONE', #4215, #7750, #12867, .T. ) ;
#7454=EDGE_LOOP ( 'NONE', ( #4188, #7251, #6313, #9306 ) ) ;
#7455=CARTESIAN_POINT ( 'NONE',  ( 2.500000000000001776, 64.00000000000000000, 49.99999999999999289 ) ) ;
#7463=CARTESIAN_POINT ( 'NONE',  ( -2.500000000000001776, 64.00000000000000000, 49.99999999999999289 ) ) ;
#7471=CARTESIAN_POINT ( 'NONE',  ( 1.461580736456473684, 65.46158073645646880, 46.05000000109246372 ) ) ;
#7480=DIRECTION ( 'NONE',  ( 0.000000000000000000, 0.000000000000000000, 1.000000000000000000 ) ) ;
#7483=CARTESIAN_POINT ( 'NONE',  ( 0.8561741729129471734, 61.93301270000000613, 46.00000000109246656 ) ) ;
#7489=VECTOR ( 'NONE', #1264, 1000.000000000000000 ) ;
#7491=( BOUNDED_CURVE ( )  B_SPLINE_CURVE ( 2, ( #1824, #10731, #18301, #7609, #16727, #1363, #2824, #16630, #15348 ),
 .UNSPECIFIED., .F., .F. ) 
 B_SPLINE_CURVE_WITH_KNOTS ( ( 3, 2, 2, 2, 3 ),
 ( 0.7142857142857141906, 0.7321428571428569843, 0.7500000000000000000, 0.7678571428571429047, 0.7857142857142856984 ),
 .UNSPECIFIED. ) 
 CURVE ( )  GEOMETRIC_REPRESENTATION_ITEM ( )  RATIONAL_B_SPLINE_CURVE ( ( 1.000000000000000444, 0.9238795325112862944, 1.000000000000000000, 0.9238795325112867385, 1.000000000000000000, 0.9238795325112867385, 1.000000000000000000, 0.9238795325112867385, 1.000000000000000000 ) ) 
 REPRESENTATION_ITEM ( '' )  );
#7495=CARTESIAN_POINT ( 'NONE',  ( -1.035533905932738641, 66.50000000000000000, 49.15000000218494591 ) ) ;
#7498=CARTESIAN_POINT ( 'NONE',  ( -1.461580736456473462, 62.53841926354353120, 45.05000000109246372 ) ) ;
#7506=DIRECTION ( 'NONE',  ( 0.000000000000000000, 0.000000000000000000, 1.000000000000000000 ) ) ;
#7511=CARTESIAN_POINT ( 'NONE',  ( 0.000000000000000000, 52.00000000000000711, -50.00000000000000000 ) ) ;
#7514=ORIENTED_EDGE ( 'NONE', *, *, #8104, .T. ) ;
#7524=DIRECTION ( 'NONE',  ( 0.000000000000000000, 0.000000000000000000, 1.000000000000000000 ) ) ;
#7530=DIRECTION ( 'NONE',  ( 0.000000000000000000, 0.000000000000000000, 1.000000000000000000 ) ) ;
#7562=CARTESIAN_POINT ( 'NONE',  ( -24.00000000000000000, 52.00000000000000711, -50.00000000000000000 ) ) ;
#7568=AXIS2_PLACEMENT_3D ( 'NONE', #16979, #6584, #1975 ) ;
#7572=EDGE_CURVE ( 'NONE', #292, #18125, #2753, .T. ) ;
#7581=CYLINDRICAL_SURFACE ( 'NONE', #2816, 2.500000000000001776 ) ;
#7583=CARTESIAN_POINT ( 'NONE',  ( 0.000000000000000000, 64.00000000000000000, 49.99999999999999289 ) ) ;
#7586=EDGE_CURVE ( 'NONE', #7101, #3717, #6879, .T. ) ;
#7590=CARTESIAN_POINT ( 'NONE',  ( 2.066987300000001859, 63.14382582708704916, 45.30000000109246372 ) ) ;
#7601=EDGE_CURVE ( 'NONE', #4696, #13296, #5354, .T. ) ;
#7603=CARTESIAN_POINT ( 'NONE',  ( 0.8561741729129472844, 61.93301270000000613, 45.20000000109248361 ) ) ;
#7609=CARTESIAN_POINT ( 'NONE',  ( -1.035533905932738641, 66.50000000000000000, 45.84999999999998721 ) ) ;
#7610=EDGE_CURVE ( 'NONE', #16061, #17639, #10872, .T. ) ;
#7611=CARTESIAN_POINT ( 'NONE',  ( -1.265664690411616068E-16, 66.06698730000000808, 47.15000000109247225 ) ) ;
#7617=( BOUNDED_CURVE ( )  B_SPLINE_CURVE ( 2, ( #490, #9500, #4820, #7652, #3531, #583, #3239, #295, #12147, #13913, #13718, #203, #15295, #5008, #12345, #15105, #7754, #12443, #13821, #3341, #15489, #1771, #16770, #1675, #6575, #2058, #6282, #5110, #1966, #9309, #6476, #16571, #9116, #13618, #6191, #10678, #7950, #12253, #10967, #9212, #18249, #10768, #15203, #1867, #7853, #399, #6382, #18343, #4913, #16867, #3430, #9403, #15397, #11405, #9932, #15650, #6727, #14459, #837, #2402, #5260, #11500, #745, #3789, #2219, #17401, #17220, #3688, #18782, #8482, #15838, #18602, #11214, #15929, #17312, #6818, #12975, #15748, #9756, #2311, #931, #18973, #8295, #4066, #5447, #12785, #3975, #17490, #1032, #2592, #16033, #12608, #2493, #14267, #7006, #11128, #5358, #8573, #9658, #5544, #10034 ),
 .UNSPECIFIED., .F., .F. ) 
 B_SPLINE_CURVE_WITH_KNOTS ( ( 3, 2, 2, 2, 2, 2, 2, 2, 2, 2, 2, 2, 2, 2, 2, 2, 2, 2, 2, 2, 2, 2, 2, 2, 2, 2, 2, 2, 2, 2, 2, 2, 2, 2, 2, 2, 2, 2, 2, 2, 2, 2, 2, 2, 2, 2, 2, 2, 2, 2, 3 ),
 ( 0.000000000000000000, 0.01785714285714285615, 0.03571428571428571230, 0.05357142857142856845, 0.07142857142857142461, 0.08928571428571428770, 0.1071428571428571369, 0.1250000000000000000, 0.1428571428571428492, 0.1607142857142857262, 0.1785714285714285754, 0.1964285714285714246, 0.2142857142857142738, 0.2321428571428571508, 0.2500000000000000000, 0.2678571428571428492, 0.2857142857142856984, 0.3035714285714285476, 0.3214285714285714524, 0.3392857142857143016, 0.3571428571428571508, 0.3750000000000000000, 0.3928571428571428492, 0.4107142857142856984, 0.4285714285714285476, 0.4464285714285714524, 0.4642857142857143016, 0.4821428571428571508, 0.5000000000000000000, 0.5178571428571429047, 0.5357142857142856984, 0.5535714285714286031, 0.5714285714285713969, 0.5892857142857143016, 0.6071428571428570953, 0.6250000000000000000, 0.6428571428571429047, 0.6607142857142856984, 0.6785714285714286031, 0.6964285714285715079, 0.7142857142857143016, 0.7321428571428570953, 0.7500000000000000000, 0.7678571428571429047, 0.7857142857142856984, 0.8035714285714286031, 0.8214285714285713969, 0.8392857142857143016, 0.8571428571428570953, 0.8750000000000000000, 0.8928571428571429047 ),
 .UNSPECIFIED. ) 
 CURVE ( )  GEOMETRIC_REPRESENTATION_ITEM ( )  RATIONAL_B_SPLINE_CURVE ( ( 1.000000000000000000, 0.9238795325112867385, 1.000000000000000000, 0.9238795325112867385, 1.000000000000000000, 0.9238795325112867385, 1.000000000000000000, 0.9238795325112867385, 1.000000000000000000, 0.9238795325112867385, 1.000000000000000000, 0.9238795325112867385, 1.000000000000000000, 0.9238795325112867385, 1.000000000000000000, 0.9238795325112867385, 1.000000000000000000, 0.9238795325112867385, 1.000000000000000000, 0.9238795325112867385, 1.000000000000000000, 0.9238795325112867385, 1.000000000000000000, 0.9238795325112867385, 1.000000000000000000, 0.9238795325112867385, 1.000000000000000000, 0.9238795325112867385, 1.000000000000000000, 0.9238795325112867385, 1.000000000000000000, 0.9238795325112867385, 1.000000000000000000, 0.9238795325112867385, 1.000000000000000000, 0.9238795325112867385, 1.000000000000000000, 0.9238795325112867385, 1.000000000000000000, 0.9238795325112867385, 1.000000000000000000, 0.9238795325112867385, 1.000000000000000000, 0.9238795325112867385, 1.000000000000000000, 0.9238795325112867385, 1.000000000000000000, 0.9238795325112867385, 1.000000000000000000, 0.9238795325112867385, 1.000000000000000000, 0.9238795325112867385, 1.000000000000000000, 0.9238795325112867385, 1.000000000000000000, 0.9238795325112867385, 1.000000000000000000, 0.9238795325112867385, 1.000000000000000000, 0.9238795325112867385, 1.000000000000000000, 0.9238795325112867385, 1.000000000000000000, 0.9238795325112867385, 1.000000000000000000, 0.9238795325112867385, 1.000000000000000000, 0.9238795325112867385, 1.000000000000000000, 0.9238795325112867385, 1.000000000000000000, 0.9238795325112867385, 1.000000000000000000, 0.9238795325112867385, 1.000000000000000000, 0.9238795325112867385, 1.000000000000000000, 0.9238795325112867385, 1.000000000000000000, 0.9238795325112867385, 1.000000000000000000, 0.9238795325112867385, 1.000000000000000000, 0.9238795325112867385, 1.000000000000000000, 0.9238795325112867385, 1.000000000000000000, 0.9238795325112867385, 1.000000000000000000, 0.9238795325112867385, 1.000000000000000000, 0.9238795325112867385, 1.000000000000000000, 0.9238795325112867385, 1.000000000000000000, 0.9238795325112867385, 1.000000000000000000, 0.9238795325112867385, 1.000000000000000000, 0.9238795325112867385, 1.000000000000000000 ) ) 
 REPRESENTATION_ITEM ( '' )  );
#7627=CARTESIAN_POINT ( 'NONE',  ( -2.066987300000001415, 64.00000000000000000, 49.55000000109247082 ) ) ;
#7629=CARTESIAN_POINT ( 'NONE',  ( -1.461580736456473462, 62.53841926354353120, 48.05000000109247082 ) ) ;
#7635=ORIENTED_EDGE ( 'NONE', *, *, #9137, .T. ) ;
#7643=ORIENTED_EDGE ( 'NONE', *, *, #16772, .F. ) ;
#7646=DIRECTION ( 'NONE',  ( 1.000000000000000000, 0.000000000000000000, 0.000000000000000000 ) ) ;
#7651=AXIS2_PLACEMENT_3D ( 'NONE', #10717, #434, #10809 ) ;
#7652=CARTESIAN_POINT ( 'NONE',  ( -0.8561741729129461742, 66.06698730000000808, 49.40000000109247225 ) ) ;
#7664=CARTESIAN_POINT ( 'NONE',  ( 2.500000000000001776, 64.00000000000000000, 48.90000000218494591 ) ) ;
#7675=CARTESIAN_POINT ( 'NONE',  ( 0.000000000000000000, 0.000000000000000000, -50.00000000000000000 ) ) ;
#7686=CARTESIAN_POINT ( 'NONE',  ( 2.066987300000001415, 64.00000000000000000, 47.75000000109246656 ) ) ;
#7687=EDGE_CURVE ( 'NONE', #2714, #13223, #13170, .T. ) ;
#7697=CARTESIAN_POINT ( 'NONE',  ( -2.500000000000001776, 64.00000000000000000, 48.50000000218494023 ) ) ;
#7700=CARTESIAN_POINT ( 'NONE',  ( -2.066987300000001859, 64.85617417291294373, 44.90000000109247225 ) ) ;
#7703=VECTOR ( 'NONE', #15478, 1000.000000000000000 ) ;
#7708=CARTESIAN_POINT ( 'NONE',  ( -2.066987300000001415, 64.00000000000000000, 46.55000000109247082 ) ) ;
#7726=ORIENTED_EDGE ( 'NONE', *, *, #6706, .T. ) ;
#7730=CARTESIAN_POINT ( 'NONE',  ( 2.066987300000001415, 64.00000000000000000, 48.35000000109246798 ) ) ;
#7733=EDGE_LOOP ( 'NONE', ( #18432, #5791, #1993, #2105 ) ) ;
#7747=VERTEX_POINT ( 'NONE', #7562 ) ;
#7750=VERTEX_POINT ( 'NONE', #14920 ) ;
#7753=STYLED_ITEM ( 'NONE', ( #17513 ), #1517 ) ;
#7754=CARTESIAN_POINT ( 'NONE',  ( -2.066987300000001415, 64.00000000000000000, 48.75000000109246656 ) ) ;
#7769=CARTESIAN_POINT ( 'NONE',  ( 2.500000000000001776, 64.00000000000000000, 48.10000000218494165 ) ) ;
#7788=DIRECTION ( 'NONE',  ( -1.000000000000000000, 0.000000000000000000, 0.000000000000000000 ) ) ;
#7795=CARTESIAN_POINT ( 'NONE',  ( 1.767766952966370653, 62.23223304703363112, 45.60000000218494165 ) ) ;
#7802=DIRECTION ( 'NONE',  ( 0.000000000000000000, 0.000000000000000000, -1.000000000000000000 ) ) ;
#7804=CARTESIAN_POINT ( 'NONE',  ( -2.066987300000001415, 63.14382582708705627, 49.00000000109246656 ) ) ;
#7806=AXIS2_PLACEMENT_3D ( 'NONE', #9461, #13970, #543 ) ;
#7810=EDGE_CURVE ( 'NONE', #9430, #15274, #17861, .T. ) ;
#7829=ORIENTED_EDGE ( 'NONE', *, *, #1701, .F. ) ;
#7830=DIRECTION ( 'NONE',  ( 0.000000000000000000, 0.000000000000000000, -1.000000000000000000 ) ) ;
#7844=VERTEX_POINT ( 'NONE', #215 ) ;
#7849=STYLED_ITEM ( 'NONE', ( #5314 ), #3741 ) ;
#7853=CARTESIAN_POINT ( 'NONE',  ( 3.796994071234847710E-16, 61.93301269999999903, 47.35000000109246798 ) ) ;
#7857=VECTOR ( 'NONE', #787, 1000.000000000000000 ) ;
#7865=FACE_OUTER_BOUND ( 'NONE', #10697, .T. ) ;
#7870=CARTESIAN_POINT ( 'NONE',  ( -2.500000000000001776, 65.03553390593273775, 49.25000000218494023 ) ) ;
#7877=AXIS2_PLACEMENT_3D ( 'NONE', #17414, #11512, #6929 ) ;
#7881=EDGE_CURVE ( 'NONE', #16382, #8256, #1784, .T. ) ;
#7889=DIRECTION ( 'NONE',  ( 0.000000000000000000, 0.000000000000000000, -1.000000000000000000 ) ) ;
#7896=DIRECTION ( 'NONE',  ( 0.000000000000000000, -1.000000000000000000, 0.000000000000000000 ) ) ;
#7899=AXIS2_PLACEMENT_3D ( 'NONE', #12103, #12306, #16825 ) ;
#7902=CARTESIAN_POINT ( 'NONE',  ( 2.500000000000002220, 62.96446609406726935, 47.25000000218494023 ) ) ;
#7910=CARTESIAN_POINT ( 'NONE',  ( -0.8561741729129465073, 61.93301270000000613, 47.50000000109246656 ) ) ;
#7913=VECTOR ( 'NONE', #4962, 1000.000000000000000 ) ;
#7915=FACE_OUTER_BOUND ( 'NONE', #12080, .T. ) ;
#7927=CARTESIAN_POINT ( 'NONE',  ( -2.066987300000001415, 64.00000000000000000, 47.95000000109246940 ) ) ;
#7929=ORIENTED_EDGE ( 'NONE', *, *, #15942, .T. ) ;
#7950=CARTESIAN_POINT ( 'NONE',  ( -1.265664690411616068E-16, 66.06698730000000808, 47.75000000109246656 ) ) ;
#7961=DIRECTION ( 'NONE',  ( 0.000000000000000000, 0.000000000000000000, 1.000000000000000000 ) ) ;
#7969=ORIENTED_EDGE ( 'NONE', *, *, #16089, .F. ) ;
#7980=CARTESIAN_POINT ( 'NONE',  ( -2.066987300000001415, 64.00000000000000000, 49.65000000109247225 ) ) ;
#7983=CARTESIAN_POINT ( 'NONE',  ( -1.767766952966369765, 62.23223304703363112, 46.09999999999999432 ) ) ;
#7992=LINE ( 'NONE', #6703, #6465 ) ;
#7997=CARTESIAN_POINT ( 'NONE',  ( -2.500000000000000888, 62.96446609406726935, 46.95000000218495018 ) ) ;
#8005=CARTESIAN_POINT ( 'NONE',  ( -2.066987300000001415, 64.00000000000000000, 47.35000000109246798 ) ) ;
#8021=LINE ( 'NONE', #4983, #8024 ) ;
#8023=AXIS2_PLACEMENT_3D ( 'NONE', #17938, #10267, #17540 ) ;
#8024=VECTOR ( 'NONE', #9373, 1000.000000000000000 ) ;
#8025=CARTESIAN_POINT ( 'NONE',  ( 1.461580736456473906, 62.53841926354353120, 47.45000000109246940 ) ) ;
#8054=ORIENTED_EDGE ( 'NONE', *, *, #15942, .F. ) ;
#8079=EDGE_LOOP ( 'NONE', ( #7121, #16567, #4547, #13033 ) ) ;
#8092=CARTESIAN_POINT ( 'NONE',  ( 1.035533905932739751, 61.50000000000000000, 47.15000000218494591 ) ) ;
#8101=CARTESIAN_POINT ( 'NONE',  ( 0.8561741729129460632, 66.06698729999999387, 45.50000000109247367 ) ) ;
#8102=DIRECTION ( 'NONE',  ( 0.000000000000000000, 1.000000000000000000, 0.000000000000000000 ) ) ;
#8104=EDGE_CURVE ( 'NONE', #10386, #3710, #14885, .T. ) ;
#8114=AXIS2_PLACEMENT_3D ( 'NONE', #698, #9415, #18642 ) ;
#8115=CARTESIAN_POINT ( 'NONE',  ( -1.265664690411616068E-16, 66.06698730000000808, 47.75000000109246656 ) ) ;
#8122=LINE ( 'NONE', #1847, #16892 ) ;
#8123=LINE ( 'NONE', #18329, #3112 ) ;
#8135=ORIENTED_EDGE ( 'NONE', *, *, #15515, .T. ) ;
#8139=CARTESIAN_POINT ( 'NONE',  ( -1.035533905932738641, 66.50000000000000000, 47.44999999999998863 ) ) ;
#8141=CARTESIAN_POINT ( 'NONE',  ( -15.00000000000000000, 35.00000000000000000, 0.000000000000000000 ) ) ;
#8163=VECTOR ( 'NONE', #2134, 1000.000000000000000 ) ;
#8166=CARTESIAN_POINT ( 'NONE',  ( 1.767766952966369987, 65.76776695296638309, 45.69999999999999574 ) ) ;
#8182=DIRECTION ( 'NONE',  ( 0.000000000000000000, 9.912705577010328508E-16, 1.000000000000000000 ) ) ;
#8183=DIRECTION ( 'NONE',  ( 0.000000000000000000, 1.000000000000000000, 0.000000000000000000 ) ) ;
#8190=CARTESIAN_POINT ( 'NONE',  ( -1.035533905932738641, 66.50000000000000000, 44.35000000218493454 ) ) ;
#8197=CARTESIAN_POINT ( 'NONE',  ( 0.000000000000000000, 64.00000000000000000, 49.99999999999999289 ) ) ;
#8202=CARTESIAN_POINT ( 'NONE',  ( -1.035533905932738863, 61.50000000000000000, 48.54999999999999716 ) ) ;
#8207=LINE ( 'NONE', #5073, #10165 ) ;
#8215=ADVANCED_FACE ( 'NONE', ( #11709, #68 ), #159, .T. ) ;
#8217=CARTESIAN_POINT ( 'NONE',  ( 2.066987300000001415, 64.00000000000000000, 47.55000000109247082 ) ) ;
#8221=AXIS2_PLACEMENT_3D ( 'NONE', #8576, #11408, #1126 ) ;
#8256=VERTEX_POINT ( 'NONE', #13380 ) ;
#8269=CARTESIAN_POINT ( 'NONE',  ( 2.500000000000001776, 64.00000000000000000, 45.70000000218494307 ) ) ;
#8274=UNCERTAINTY_MEASURE_WITH_UNIT (LENGTH_MEASURE( 1.000000000000000082E-05 ), #12904, 'distance_accuracy_value', 'NONE');
#8277=CARTESIAN_POINT ( 'NONE',  ( 2.066987300000001859, 64.85617417291294373, 46.80000000109246372 ) ) ;
#8284=CARTESIAN_POINT ( 'NONE',  ( -24.00000000000000000, 47.00000000000000711, -50.00000000000000000 ) ) ;
#8286=CARTESIAN_POINT ( 'NONE',  ( -1.461580736456473462, 62.53841926354353120, 45.05000000109246372 ) ) ;
#8295=CARTESIAN_POINT ( 'NONE',  ( -1.461580736456473906, 65.46158073645646880, 45.45000000109246940 ) ) ;
#8297=PLANE ( 'NONE',  #999 ) ;
#8299=CARTESIAN_POINT ( 'NONE',  ( 0.8561741729129460632, 66.06698729999999387, 45.30000000109247082 ) ) ;
#8309=CARTESIAN_POINT ( 'NONE',  ( 32.50000000000000000, 52.00000000000000711, 15.00000000000000000 ) ) ;
#8313=ORIENTED_EDGE ( 'NONE', *, *, #958, .T. ) ;
#8316=SHAPE_REPRESENTATION_RELATIONSHIP ( 'NONE' , 'NONE' ,  #12005, #1517 ) ;
#8326=EDGE_LOOP ( 'NONE', ( #2967, #18535, #1833, #15792 ) ) ;
#8328=ORIENTED_EDGE ( 'NONE', *, *, #4349, .T. ) ;
#8330=ORIENTED_EDGE ( 'NONE', *, *, #14647, .T. ) ;
#8344=CARTESIAN_POINT ( 'NONE',  ( -2.500000000000001776, 64.00000000000000000, 49.30000000218494449 ) ) ;
#8352=CARTESIAN_POINT ( 'NONE',  ( -15.00000000000000000, 47.00000000000000711, 30.00000000000000000 ) ) ;
#8359=CARTESIAN_POINT ( 'NONE',  ( 1.767766952966370653, 62.23223304703363112, 48.00000000218494023 ) ) ;
#8369=CARTESIAN_POINT ( 'NONE',  ( 1.461580736456473684, 65.46158073645646880, 48.45000000109247651 ) ) ;
#8378=CARTESIAN_POINT ( 'NONE',  ( 1.767766952966370653, 62.23223304703363112, 49.49999999999999289 ) ) ;
#8388=CARTESIAN_POINT ( 'NONE',  ( -0.8561741729129461742, 66.06698729999999387, 44.60000000109246088 ) ) ;
#8390=LINE ( 'NONE', #9573, #8163 ) ;
#8401=ORIENTED_EDGE ( 'NONE', *, *, #6076, .T. ) ;
#8404=VERTEX_POINT ( 'NONE', #12206 ) ;
#8413=ORIENTED_EDGE ( 'NONE', *, *, #7687, .T. ) ;
#8414=EDGE_CURVE ( 'NONE', #18580, #7844, #9361, .T. ) ;
#8415=DIRECTION ( 'NONE',  ( 0.000000000000000000, 0.000000000000000000, 1.000000000000000000 ) ) ;
#8426=CARTESIAN_POINT ( 'NONE',  ( -2.500000000000001776, 64.00000000000000000, 49.99999999999999289 ) ) ;
#8431=LINE ( 'NONE', #17269, #4622 ) ;
#8441=VECTOR ( 'NONE', #730, 1000.000000000000000 ) ;
#8444=VECTOR ( 'NONE', #9294, 1000.000000000000000 ) ;
#8450=CARTESIAN_POINT ( 'NONE',  ( 2.500000000000001776, 64.00000000000000000, 48.10000000218494165 ) ) ;
#8462=CARTESIAN_POINT ( 'NONE',  ( 2.066987300000001859, 64.85617417291294373, 47.60000000109246798 ) ) ;
#8466=PLANE ( 'NONE',  #15012 ) ;
#8470=AXIS2_PLACEMENT_3D ( 'NONE', #4510, #13705, #10370 ) ;
#8473=CARTESIAN_POINT ( 'NONE',  ( 1.461580736456473906, 62.53841926354353120, 45.25000000109247367 ) ) ;
#8474=CARTESIAN_POINT ( 'NONE',  ( 1.461580736456473906, 62.53841926354353120, 49.25000000109246656 ) ) ;
#8480=ORIENTED_EDGE ( 'NONE', *, *, #15119, .T. ) ;
#8482=CARTESIAN_POINT ( 'NONE',  ( 0.8561741729129460632, 66.06698730000000808, 46.10000000109246798 ) ) ;
#8486=CARTESIAN_POINT ( 'NONE',  ( 2.066987300000001859, 64.85617417291294373, 49.40000000109246514 ) ) ;
#8492=LINE ( 'NONE', #5553, #9991 ) ;
#8507=DIRECTION ( 'NONE',  ( -0.000000000000000000, -0.000000000000000000, -1.000000000000000000 ) ) ;
#8509=CARTESIAN_POINT ( 'NONE',  ( 0.000000000000000000, 0.000000000000000000, 30.00000000000000000 ) ) ;
#8512=DIRECTION ( 'NONE',  ( -0.000000000000000000, -0.000000000000000000, -1.000000000000000000 ) ) ;
#8515=EDGE_LOOP ( 'NONE', ( #6209, #18236, #3923, #6362 ) ) ;
#8518=DIRECTION ( 'NONE',  ( -0.000000000000000000, -1.000000000000000000, 0.000000000000000000 ) ) ;
#8531=CIRCLE ( 'NONE', #18575, 2.499999999999998668 ) ;
#8534=CARTESIAN_POINT ( 'NONE',  ( 2.500000000000002220, 62.96446609406726935, 45.54999999999999716 ) ) ;
#8547=ADVANCED_FACE ( 'NONE', ( #5711 ), #6718, .T. ) ;
#8555=CARTESIAN_POINT ( 'NONE',  ( 2.066987300000001859, 64.85617417291294373, 48.40000000109247225 ) ) ;
#8564=EDGE_CURVE ( 'NONE', #297, #13006, #11121, .T. ) ;
#8566=CARTESIAN_POINT ( 'NONE',  ( -2.500000000000001776, 64.00000000000000000, 47.59999999999999432 ) ) ;
#8567=CARTESIAN_POINT ( 'NONE',  ( -1.767766952966369765, 62.23223304703363112, 49.29999999999999716 ) ) ;
#8568=CARTESIAN_POINT ( 'NONE',  ( 24.00000000000000000, 52.00000000000000711, -67.72004514666936359 ) ) ;
#8573=CARTESIAN_POINT ( 'NONE',  ( -2.066987300000001415, 64.85617417291294373, 44.70000000109248361 ) ) ;
#8576=CARTESIAN_POINT ( 'NONE',  ( -4.000000000000001776, 67.00000000000000000, 34.99999999999999289 ) ) ;
#8578=CARTESIAN_POINT ( 'NONE',  ( 0.8561741729129472844, 61.93301270000000613, 49.20000000109247651 ) ) ;
#8588=CARTESIAN_POINT ( 'NONE',  ( -2.500000000000001776, 64.00000000000000000, 48.39999999999999858 ) ) ;
#8593=ORIENTED_EDGE ( 'NONE', *, *, #3737, .T. ) ;
#8628=PLANE ( 'NONE',  #8788 ) ;
#8648=CARTESIAN_POINT ( 'NONE',  ( 0.8561741729129472844, 61.93301270000000613, 48.20000000109248361 ) ) ;
#8651=ORIENTED_EDGE ( 'NONE', *, *, #2594, .F. ) ;
#8655=EDGE_CURVE ( 'NONE', #8882, #2308, #11669, .T. ) ;
#8661=CARTESIAN_POINT ( 'NONE',  ( -2.500000000000001776, 65.03553390593273775, 46.74999999999999289 ) ) ;
#8662=CARTESIAN_POINT ( 'NONE',  ( -0.8561741729129461742, 66.06698730000000808, 48.80000000109247082 ) ) ;
#8663=CARTESIAN_POINT ( 'NONE',  ( 2.499999999999996003, 62.96446609406726225, 48.85000000218494165 ) ) ;
#8671=EDGE_CURVE ( 'NONE', #5010, #9208, #11470, .T. ) ;
#8672=CARTESIAN_POINT ( 'NONE',  ( 0.8561741729129460632, 66.06698729999999387, 49.50000000109246656 ) ) ;
#8719=VECTOR ( 'NONE', #12659, 1000.000000000000000 ) ;
#8721=ORIENTED_EDGE ( 'NONE', *, *, #1701, .T. ) ;
#8727=CARTESIAN_POINT ( 'NONE',  ( -1.265664690411616068E-16, 66.06698730000000808, 44.55000000109247082 ) ) ;
#8733=DIRECTION ( 'NONE',  ( -1.000000000000000000, 0.000000000000000000, 0.000000000000000000 ) ) ;
#8736=VECTOR ( 'NONE', #11000, 1000.000000000000000 ) ;
#8739=CARTESIAN_POINT ( 'NONE',  ( -2.066987300000001415, 63.14382582708705627, 45.60000000109246088 ) ) ;
#8748=EDGE_CURVE ( 'NONE', #6376, #16061, #16900, .T. ) ;
#8753=CARTESIAN_POINT ( 'NONE',  ( -1.767766952966370209, 65.76776695296638309, 47.49999999999999289 ) ) ;
#8754=CARTESIAN_POINT ( 'NONE',  ( -0.8561741729129461742, 66.06698730000000808, 48.00000000109246656 ) ) ;
#8766=CARTESIAN_POINT ( 'NONE',  ( -1.035533905932738641, 66.50000000000000000, 48.35000000218494165 ) ) ;
#8769=CARTESIAN_POINT ( 'NONE',  ( -1.461580736456473462, 62.53841926354353120, 49.05000000109247082 ) ) ;
#8773=CARTESIAN_POINT ( 'NONE',  ( -1.265664690411616068E-16, 66.06698730000000808, 49.55000000109247082 ) ) ;
#8778=DIRECTION ( 'NONE',  ( 0.000000000000000000, 0.000000000000000000, 1.000000000000000000 ) ) ;
#8788=AXIS2_PLACEMENT_3D ( 'NONE', #7158, #15801, #14709 ) ;
#8795=DIRECTION ( 'NONE',  ( 1.000000000000000000, 0.000000000000000000, 0.000000000000000000 ) ) ;
#8813=VECTOR ( 'NONE', #6634, 1000.000000000000000 ) ;
#8817=ORIENTED_EDGE ( 'NONE', *, *, #15174, .F. ) ;
#8822=ORIENTED_EDGE ( 'NONE', *, *, #16910, .T. ) ;
#8830=ORIENTED_EDGE ( 'NONE', *, *, #18890, .F. ) ;
#8832=ORIENTED_EDGE ( 'NONE', *, *, #14412, .T. ) ;
#8837=DIRECTION ( 'NONE',  ( -0.000000000000000000, -0.000000000000000000, -1.000000000000000000 ) ) ;
#8841=DIRECTION ( 'NONE',  ( 0.000000000000000000, 1.000000000000000000, -9.912705577010328508E-16 ) ) ;
#8854=CARTESIAN_POINT ( 'NONE',  ( 2.500000000000001776, 65.03553390593273775, 44.95000000218495018 ) ) ;
#8857=CARTESIAN_POINT ( 'NONE',  ( -1.530808498934192803E-16, 66.50000000000000000, 48.19999999999999574 ) ) ;
#8858=CARTESIAN_POINT ( 'NONE',  ( -1.265664690411616068E-16, 66.06698730000000808, 47.95000000109246940 ) ) ;
#8863=( BOUNDED_SURFACE ( )  B_SPLINE_SURFACE ( 1, 2, ( 
 ( #13077, #1533, #19175, #15061, #8773, #16426, #8972, #14959, #1825, #18498, #12204, #10629, #9358, #3582, #3298, #7804, #9268, #156, #15254, #17025, #1726, #18402, #450, #13974, #13776, #6436, #16729, #1928, #12307, #16632, #18303, #356, #6342, #9554, #5067, #12497, #4968, #1638, #546, #6144, #16926, #2016, #4871, #6531, #10832, #7910, #11023, #16827, #8005, #3389, #6238, #15349, #7611, #15449, #18206, #13875, #4782, #12404, #3199, #10925, #3488, #13575, #9173, #15158, #7708, #12104, #9463, #18101, #10733, #4673, #13674, #253, #5157, #5347, #15826, #17116, #14069, #9833, #5441, #18590, #17390, #642, #12878, #2209, #6904, #8101, #737, #15740, #6632, #5534, #8473, #6716, #18963, #921, #8286, #18877, #12967, #15922, #17480, #11492, #12599 ),
 ( #17211, #4058, #11118, #3965, #6999, #15637, #3679, #17305, #15547, #11309, #8378, #9748, #6811, #3867, #12777, #11396, #12686, #2393, #11206, #2484, #3778, #14348, #18690, #9650, #5254, #14449, #18772, #9924, #1025, #8202, #14168, #2302, #2117, #14256, #829, #17681, #8857, #19056, #7189, #13060, #5629, #2776, #7096, #4166, #4359, #13259, #1320, #10116, #8566, #2879, #8753, #7292, #14544, #16115, #14742, #16025, #4259, #2680, #19257, #5825, #11591, #10023, #11791, #14842, #17589, #8661, #17783, #14641, #10315, #2584, #1115, #13163, #7388, #1414, #1208, #19160, #5731, #11690, #10220, #16209, #16311, #5496, #15708, #11364, #12933, #11273, #8166, #5227, #4022, #8534, #2364, #14508, #6692, #1079, #7057, #5409, #2276, #11181, #9898, #13028, #11554 ) ),
 .UNSPECIFIED., .F., .F., .F. ) 
 B_SPLINE_SURFACE_WITH_KNOTS ( ( 2, 2 ),
 ( 3, 2, 2, 2, 2, 2, 2, 2, 2, 2, 2, 2, 2, 2, 2, 2, 2, 2, 2, 2, 2, 2, 2, 2, 2, 2, 2, 2, 2, 2, 2, 2, 2, 2, 2, 2, 2, 2, 2, 2, 2, 2, 2, 2, 2, 2, 2, 2, 2, 2, 3 ),
 ( 0.000000000000000000, 1.000000000000000000 ),
 ( 0.000000000000000000, 0.01785714285714285615, 0.03571428571428571230, 0.05357142857142856845, 0.07142857142857142461, 0.08928571428571428770, 0.1071428571428571369, 0.1250000000000000000, 0.1428571428571428492, 0.1607142857142857262, 0.1785714285714285754, 0.1964285714285714246, 0.2142857142857142738, 0.2321428571428571508, 0.2500000000000000000, 0.2678571428571428492, 0.2857142857142856984, 0.3035714285714285476, 0.3214285714285714524, 0.3392857142857143016, 0.3571428571428571508, 0.3750000000000000000, 0.3928571428571428492, 0.4107142857142856984, 0.4285714285714285476, 0.4464285714285714524, 0.4642857142857143016, 0.4821428571428571508, 0.5000000000000000000, 0.5178571428571429047, 0.5357142857142856984, 0.5535714285714286031, 0.5714285714285713969, 0.5892857142857143016, 0.6071428571428570953, 0.6250000000000000000, 0.6428571428571429047, 0.6607142857142856984, 0.6785714285714286031, 0.6964285714285713969, 0.7142857142857143016, 0.7321428571428570953, 0.7500000000000000000, 0.7678571428571429047, 0.7857142857142856984, 0.8035714285714286031, 0.8214285714285713969, 0.8392857142857143016, 0.8571428571428570953, 0.8750000000000000000, 0.8928571428571429047 ),
 .UNSPECIFIED. ) 
 GEOMETRIC_REPRESENTATION_ITEM ( )  RATIONAL_B_SPLINE_SURFACE ( (
 ( 1.000000000000000000, 0.9238795325112867385, 1.000000000000000000, 0.9238795325112867385, 1.000000000000000000, 0.9238795325112867385, 1.000000000000000000, 0.9238795325112867385, 1.000000000000000000, 0.9238795325112867385, 1.000000000000000000, 0.9238795325112867385, 1.000000000000000000, 0.9238795325112867385, 1.000000000000000000, 0.9238795325112867385, 1.000000000000000000, 0.9238795325112867385, 1.000000000000000000, 0.9238795325112867385, 1.000000000000000000, 0.9238795325112867385, 1.000000000000000000, 0.9238795325112867385, 1.000000000000000000, 0.9238795325112867385, 1.000000000000000000, 0.9238795325112867385, 1.000000000000000000, 0.9238795325112867385, 1.000000000000000000, 0.9238795325112867385, 1.000000000000000000, 0.9238795325112867385, 1.000000000000000000, 0.9238795325112867385, 1.000000000000000000, 0.9238795325112867385, 1.000000000000000000, 0.9238795325112867385, 1.000000000000000000, 0.9238795325112867385, 1.000000000000000000, 0.9238795325112867385, 1.000000000000000000, 0.9238795325112867385, 1.000000000000000000, 0.9238795325112867385, 1.000000000000000000, 0.9238795325112867385, 1.000000000000000000, 0.9238795325112867385, 1.000000000000000000, 0.9238795325112867385, 1.000000000000000000, 0.9238795325112867385, 1.000000000000000000, 0.9238795325112867385, 1.000000000000000000, 0.9238795325112867385, 1.000000000000000000, 0.9238795325112867385, 1.000000000000000000, 0.9238795325112867385, 1.000000000000000000, 0.9238795325112867385, 1.000000000000000000, 0.9238795325112867385, 1.000000000000000000, 0.9238795325112867385, 1.000000000000000000, 0.9238795325112867385, 1.000000000000000000, 0.9238795325112867385, 1.000000000000000000, 0.9238795325112867385, 1.000000000000000000, 0.9238795325112867385, 1.000000000000000000, 0.9238795325112867385, 1.000000000000000000, 0.9238795325112867385, 1.000000000000000000, 0.9238795325112867385, 1.000000000000000000, 0.9238795325112867385, 1.000000000000000000, 0.9238795325112867385, 1.000000000000000000, 0.9238795325112867385, 1.000000000000000000, 0.9238795325112867385, 1.000000000000000000, 0.9238795325112867385, 1.000000000000000000, 0.9238795325112867385, 1.000000000000000000, 0.9238795325112867385, 1.000000000000000000, 0.9238795325112867385, 1.000000000000000000),
 ( 1.000000000000000000, 0.9238795325112867385, 1.000000000000000000, 0.9238795325112867385, 1.000000000000000000, 0.9238795325112867385, 1.000000000000000000, 0.9238795325112867385, 1.000000000000000000, 0.9238795325112867385, 1.000000000000000000, 0.9238795325112867385, 1.000000000000000000, 0.9238795325112867385, 1.000000000000000000, 0.9238795325112867385, 1.000000000000000000, 0.9238795325112867385, 1.000000000000000000, 0.9238795325112867385, 1.000000000000000000, 0.9238795325112867385, 1.000000000000000000, 0.9238795325112867385, 1.000000000000000000, 0.9238795325112867385, 1.000000000000000000, 0.9238795325112867385, 1.000000000000000000, 0.9238795325112867385, 1.000000000000000000, 0.9238795325112867385, 1.000000000000000000, 0.9238795325112867385, 1.000000000000000000, 0.9238795325112867385, 1.000000000000000000, 0.9238795325112867385, 1.000000000000000000, 0.9238795325112867385, 1.000000000000000000, 0.9238795325112867385, 1.000000000000000000, 0.9238795325112867385, 1.000000000000000000, 0.9238795325112867385, 1.000000000000000000, 0.9238795325112867385, 1.000000000000000000, 0.9238795325112867385, 1.000000000000000000, 0.9238795325112867385, 1.000000000000000000, 0.9238795325112867385, 1.000000000000000000, 0.9238795325112867385, 1.000000000000000000, 0.9238795325112867385, 1.000000000000000000, 0.9238795325112867385, 1.000000000000000000, 0.9238795325112867385, 1.000000000000000000, 0.9238795325112867385, 1.000000000000000000, 0.9238795325112867385, 1.000000000000000000, 0.9238795325112867385, 1.000000000000000000, 0.9238795325112867385, 1.000000000000000000, 0.9238795325112867385, 1.000000000000000000, 0.9238795325112867385, 1.000000000000000000, 0.9238795325112867385, 1.000000000000000000, 0.9238795325112867385, 1.000000000000000000, 0.9238795325112867385, 1.000000000000000000, 0.9238795325112867385, 1.000000000000000000, 0.9238795325112867385, 1.000000000000000000, 0.9238795325112867385, 1.000000000000000000, 0.9238795325112867385, 1.000000000000000000, 0.9238795325112867385, 1.000000000000000000, 0.9238795325112867385, 1.000000000000000000, 0.9238795325112867385, 1.000000000000000000, 0.9238795325112867385, 1.000000000000000000, 0.9238795325112867385, 1.000000000000000000, 0.9238795325112867385, 1.000000000000000000) ) ) 
 REPRESENTATION_ITEM ( '' )  SURFACE ( )  );
#8867=CARTESIAN_POINT ( 'NONE',  ( -1.530808498934192803E-16, 66.50000000000000000, 49.10000000218494165 ) ) ;
#8869=CARTESIAN_POINT ( 'NONE',  ( -2.066987300000001859, 64.85617417291294373, 46.50000000109246656 ) ) ;
#8878=CARTESIAN_POINT ( 'NONE',  ( -32.50000000000000000, 52.00000000000000711, -35.00000000000000000 ) ) ;
#8882=VERTEX_POINT ( 'NONE', #10590 ) ;
#8891=CARTESIAN_POINT ( 'NONE',  ( 2.066987300000001415, 64.00000000000000000, 49.15000000109247225 ) ) ;
#8899=CIRCLE ( 'NONE', #7651, 2.500000000000002220 ) ;
#8907=ORIENTED_EDGE ( 'NONE', *, *, #15752, .F. ) ;
#8917=CARTESIAN_POINT ( 'NONE',  ( 32.50000000000000000, 47.00000000000000711, 12.50000000000000000 ) ) ;
#8924=VERTEX_POINT ( 'NONE', #6493 ) ;
#8952=CARTESIAN_POINT ( 'NONE',  ( 3.796994071234847710E-16, 61.93301269999999903, 46.75000000109246656 ) ) ;
#8965=CIRCLE ( 'NONE', #10199, 2.999999999999999112 ) ;
#8967=CARTESIAN_POINT ( 'NONE',  ( -2.066987300000001415, 63.14382582708705627, 45.00000000109246656 ) ) ;
#8972=CARTESIAN_POINT ( 'NONE',  ( 1.461580736456473684, 65.46158073645646880, 49.45000000109246940 ) ) ;
#8978=( BOUNDED_CURVE ( )  B_SPLINE_CURVE ( 2, ( #16307, #1020, #10312, #11685, #16405, #10113, #7386, #8854, #13359 ),
 .UNSPECIFIED., .F., .F. ) 
 B_SPLINE_CURVE_WITH_KNOTS ( ( 3, 2, 2, 2, 3 ),
 ( 0.7142857142857141906, 0.7321428571428569843, 0.7500000000000000000, 0.7678571428571429047, 0.7857142857142856984 ),
 .UNSPECIFIED. ) 
 CURVE ( )  GEOMETRIC_REPRESENTATION_ITEM ( )  RATIONAL_B_SPLINE_CURVE ( ( 1.000000000000000444, 0.9238795325112862944, 1.000000000000000000, 0.9238795325112867385, 1.000000000000000000, 0.9238795325112867385, 1.000000000000000000, 0.9238795325112867385, 1.000000000000000000 ) ) 
 REPRESENTATION_ITEM ( '' )  );
#8990=CARTESIAN_POINT ( 'NONE',  ( -0.8561741729129461742, 66.06698729999999387, 49.40000000109247225 ) ) ;
#8996=LINE ( 'NONE', #19101, #17889 ) ;
#8998=ORIENTED_EDGE ( 'NONE', *, *, #13265, .F. ) ;
#9007=EDGE_LOOP ( 'NONE', ( #2045, #4816, #19020, #17409 ) ) ;
#9016=DIRECTION ( 'NONE',  ( 0.000000000000000000, 0.000000000000000000, 1.000000000000000000 ) ) ;
#9019=CARTESIAN_POINT ( 'NONE',  ( -24.00000000000000000, 52.00000000000000711, -67.72004514666936359 ) ) ;
#9022=ORIENTED_EDGE ( 'NONE', *, *, #11659, .F. ) ;
#9040=CARTESIAN_POINT ( 'NONE',  ( 0.8561741729129460632, 66.06698729999999387, 45.30000000109247082 ) ) ;
#9048=CYLINDRICAL_SURFACE ( 'NONE', #6868, 2.500000000000001776 ) ;
#9050=FACE_BOUND ( 'NONE', #19086, .T. ) ;
#9052=CARTESIAN_POINT ( 'NONE',  ( 2.066987300000001415, 64.00000000000000000, 45.35000000109246798 ) ) ;
#9063=CARTESIAN_POINT ( 'NONE',  ( 4.592425496802577917E-16, 61.50000000000000000, 47.90000000218494591 ) ) ;
#9093=CARTESIAN_POINT ( 'NONE',  ( -0.8561741729129465073, 61.93301270000000613, 48.10000000109246798 ) ) ;
#9111=VECTOR ( 'NONE', #11375, 1000.000000000000000 ) ;
#9116=CARTESIAN_POINT ( 'NONE',  ( -2.066987300000001415, 64.00000000000000000, 47.95000000109246940 ) ) ;
#9121=VECTOR ( 'NONE', #15937, 1000.000000000000000 ) ;
#9132=DIRECTION ( 'NONE',  ( -0.000000000000000000, -1.000000000000000000, 0.000000000000000000 ) ) ;
#9134=CIRCLE ( 'NONE', #5691, 2.500000000000002220 ) ;
#9137=EDGE_CURVE ( 'NONE', #2714, #9379, #15696, .T. ) ;
#9140=VERTEX_POINT ( 'NONE', #6774 ) ;
#9154=CARTESIAN_POINT ( 'NONE',  ( -0.8561741729129466183, 61.93301270000000613, 46.70000000109248361 ) ) ;
#9163=CARTESIAN_POINT ( 'NONE',  ( -2.500000000000001776, 64.00000000000000000, 49.30000000218494449 ) ) ;
#9165=CARTESIAN_POINT ( 'NONE',  ( 0.8561741729129472844, 61.93301270000000613, 46.00000000109245946 ) ) ;
#9173=CARTESIAN_POINT ( 'NONE',  ( -1.461580736456473462, 62.53841926354353120, 46.65000000109247225 ) ) ;
#9181=ORIENTED_EDGE ( 'NONE', *, *, #5923, .T. ) ;
#9190=CARTESIAN_POINT ( 'NONE',  ( -2.066987300000001415, 64.00000000000000000, 48.75000000109246656 ) ) ;
#9198=DIRECTION ( 'NONE',  ( 0.8660254037844385966, 0.000000000000000000, 0.5000000000000001110 ) ) ;
#9201=CARTESIAN_POINT ( 'NONE',  ( 32.50000000000000000, 52.00000000000000711, 12.50000000000000000 ) ) ;
#9208=VERTEX_POINT ( 'NONE', #19111 ) ;
#9212=CARTESIAN_POINT ( 'NONE',  ( 2.066987300000001415, 64.85617417291294373, 47.60000000109246798 ) ) ;
#9221=CARTESIAN_POINT ( 'NONE',  ( -2.500000000000001776, 64.00000000000000000, 49.99999999999999289 ) ) ;
#9228=VECTOR ( 'NONE', #9645, 1000.000000000000000 ) ;
#9257=CARTESIAN_POINT ( 'NONE',  ( 1.767766952966369987, 65.76776695296638309, 45.00000000218494733 ) ) ;
#9260=CARTESIAN_POINT ( 'NONE',  ( 2.066987300000001415, 64.00000000000000000, 45.35000000109246798 ) ) ;
#9268=CARTESIAN_POINT ( 'NONE',  ( -2.066987300000001415, 64.00000000000000000, 48.95000000109246940 ) ) ;
#9285=CARTESIAN_POINT ( 'NONE',  ( -1.265664690411616068E-16, 66.06698730000000808, 48.55000000109247082 ) ) ;
#9294=DIRECTION ( 'NONE',  ( 1.000000000000000000, 0.000000000000000000, 0.000000000000000000 ) ) ;
#9306=ORIENTED_EDGE ( 'NONE', *, *, #8104, .F. ) ;
#9309=CARTESIAN_POINT ( 'NONE',  ( -0.8561741729129466183, 61.93301270000000613, 48.10000000109246798 ) ) ;
#9325=EDGE_LOOP ( 'NONE', ( #12329, #9582, #12463, #8593, #6690, #7929, #7514, #18431, #8328, #17816, #4619, #10639, #15683, #14990, #10388, #8651 ) ) ;
#9328=ORIENTED_EDGE ( 'NONE', *, *, #5225, .F. ) ;
#9342=EDGE_CURVE ( 'NONE', #4943, #13549, #19015, .T. ) ;
#9347=CARTESIAN_POINT ( 'NONE',  ( -2.500000000000001776, 64.00000000000000000, 46.90000000218494591 ) ) ;
#9354=AXIS2_PLACEMENT_3D ( 'NONE', #19203, #17934, #13401 ) ;
#9356=DIRECTION ( 'NONE',  ( 0.000000000000000000, 1.000000000000000000, -0.000000000000000000 ) ) ;
#9358=CARTESIAN_POINT ( 'NONE',  ( 3.796994071234847710E-16, 61.93301269999999903, 49.15000000109246514 ) ) ;
#9361=LINE ( 'NONE', #15351, #17908 ) ;
#9373=DIRECTION ( 'NONE',  ( 1.000000000000000000, 0.000000000000000000, 0.000000000000000000 ) ) ;
#9377=CARTESIAN_POINT ( 'NONE',  ( -1.461580736456473462, 62.53841926354353120, 46.45000000109246940 ) ) ;
#9379=VERTEX_POINT ( 'NONE', #9201 ) ;
#9385=DIRECTION ( 'NONE',  ( 0.000000000000000000, 1.000000000000000000, 0.000000000000000000 ) ) ;
#9403=CARTESIAN_POINT ( 'NONE',  ( -0.8561741729129461742, 66.06698730000000808, 47.00000000109247367 ) ) ;
#9414=EDGE_CURVE ( 'NONE', #4427, #12045, #652, .T. ) ;
#9415=DIRECTION ( 'NONE',  ( 0.000000000000000000, 0.000000000000000000, -1.000000000000000000 ) ) ;
#9430=VERTEX_POINT ( 'NONE', #4611 ) ;
#9440=EDGE_CURVE ( 'NONE', #18899, #9379, #16939, .T. ) ;
#9444=CARTESIAN_POINT ( 'NONE',  ( -1.035533905932738641, 66.50000000000000000, 45.95000000218494307 ) ) ;
#9453=CARTESIAN_POINT ( 'NONE',  ( 1.035533905932739751, 61.50000000000000000, 45.55000000218493739 ) ) ;
#9461=CARTESIAN_POINT ( 'NONE',  ( -32.50000000000000000, 52.00000000000000711, 15.00000000000000000 ) ) ;
#9463=CARTESIAN_POINT ( 'NONE',  ( -1.461580736456473906, 65.46158073645646880, 46.45000000109246940 ) ) ;
#9464=CARTESIAN_POINT ( 'NONE',  ( 1.035533905932739751, 61.50000000000000000, 49.44999999999999574 ) ) ;
#9478=CARTESIAN_POINT ( 'NONE',  ( -0.8561741729129465073, 61.93301270000000613, 44.90000000109247225 ) ) ;
#9495=EDGE_LOOP ( 'NONE', ( #4218, #7969, #11362, #13919, #3000 ) ) ;
#9500=CARTESIAN_POINT ( 'NONE',  ( -2.066987300000001415, 64.85617417291294373, 49.50000000109246656 ) ) ;
#9521=CARTESIAN_POINT ( 'NONE',  ( -15.00000000000000000, 47.00000000000000711, 0.000000000000000000 ) ) ;
#9527=CARTESIAN_POINT ( 'NONE',  ( -14.99999999999999645, 73.00000000000001421, 23.99999999999997868 ) ) ;
#9528=ORIENTED_EDGE ( 'NONE', *, *, #2771, .T. ) ;
#9545=CARTESIAN_POINT ( 'NONE',  ( -2.500000000000001776, 65.03553390593273775, 44.45000000218495018 ) ) ;
#9554=CARTESIAN_POINT ( 'NONE',  ( -2.066987300000001859, 64.85617417291294373, 48.10000000109246798 ) ) ;
#9569=CARTESIAN_POINT ( 'NONE',  ( -0.8561741729129465073, 61.93301270000000613, 46.50000000109247367 ) ) ;
#9573=CARTESIAN_POINT ( 'NONE',  ( 24.00000000000000000, 0.000000000000000000, -50.00000000000000000 ) ) ;
#9582=ORIENTED_EDGE ( 'NONE', *, *, #15990, .T. ) ;
#9588=ORIENTED_EDGE ( 'NONE', *, *, #15791, .F. ) ;
#9605=CARTESIAN_POINT ( 'NONE',  ( 2.500000000000001776, 64.00000000000000000, 47.99999999999999289 ) ) ;
#9617=( BOUNDED_CURVE ( )  B_SPLINE_CURVE ( 2, ( #4969, #18403, #10926, #9464, #15450, #2017, #8567, #10024, #15827 ),
 .UNSPECIFIED., .F., .F. ) 
 B_SPLINE_CURVE_WITH_KNOTS ( ( 3, 2, 2, 2, 3 ),
 ( 0.07142857142857121644, 0.08928571428571414892, 0.1071428571428570675, 0.1250000000000000000, 0.1428571428571429047 ),
 .UNSPECIFIED. ) 
 CURVE ( )  GEOMETRIC_REPRESENTATION_ITEM ( )  RATIONAL_B_SPLINE_CURVE ( ( 1.000000000000000666, 0.9238795325112857393, 1.000000000000000000, 0.9238795325112867385, 1.000000000000000000, 0.9238795325112867385, 1.000000000000000000, 0.9238795325112865164, 1.000000000000000222 ) ) 
 REPRESENTATION_ITEM ( '' )  );
#9638=ORIENTED_EDGE ( 'NONE', *, *, #9946, .T. ) ;
#9641=CARTESIAN_POINT ( 'NONE',  ( -1.767766952966370209, 65.76776695296638309, 44.40000000218493881 ) ) ;
#9643=CYLINDRICAL_SURFACE ( 'NONE', #12189, 2.500000000000001776 ) ;
#9645=DIRECTION ( 'NONE',  ( 0.000000000000000000, 1.000000000000000000, 0.000000000000000000 ) ) ;
#9650=CARTESIAN_POINT ( 'NONE',  ( 2.500000000000001776, 65.03553390593273775, 48.85000000000000142 ) ) ;
#9652=CARTESIAN_POINT ( 'NONE',  ( 1.035533905932738197, 66.50000000000000000, 48.25000000218494733 ) ) ;
#9658=CARTESIAN_POINT ( 'NONE',  ( -1.461580736456473906, 65.46158073645646880, 44.65000000109246514 ) ) ;
#9664=CARTESIAN_POINT ( 'NONE',  ( -2.066987300000001415, 63.14382582708705627, 45.60000000109246088 ) ) ;
#9676=DIRECTION ( 'NONE',  ( 0.000000000000000000, 0.000000000000000000, 1.000000000000000000 ) ) ;
#9682=VECTOR ( 'NONE', #4994, 1000.000000000000000 ) ;
#9694=ORIENTED_EDGE ( 'NONE', *, *, #18759, .F. ) ;
#9705=CIRCLE ( 'NONE', #18780, 2.499999999999998668 ) ;
#9711=VERTEX_POINT ( 'NONE', #15573 ) ;
#9729=LINE ( 'NONE', #2377, #19286 ) ;
#9735=CARTESIAN_POINT ( 'NONE',  ( 3.796994071234847710E-16, 61.93301269999999903, 46.55000000109247082 ) ) ;
#9740=CARTESIAN_POINT ( 'NONE',  ( 2.500000000000001776, 64.00000000000000000, 46.50000000218494733 ) ) ;
#9742=EDGE_CURVE ( 'NONE', #3695, #17145, #11599, .T. ) ;
#9748=CARTESIAN_POINT ( 'NONE',  ( 1.035533905932739751, 61.50000000000000000, 49.44999999999999574 ) ) ;
#9750=VECTOR ( 'NONE', #8837, 1000.000000000000000 ) ;
#9756=CARTESIAN_POINT ( 'NONE',  ( -1.461580736456473462, 62.53841926354353120, 45.65000000109247225 ) ) ;
#9758=DIRECTION ( 'NONE',  ( 0.000000000000000000, 0.000000000000000000, 1.000000000000000000 ) ) ;
#9761=CARTESIAN_POINT ( 'NONE',  ( -1.265664690411616068E-16, 66.06698730000000808, 45.35000000109246798 ) ) ;
#9769=CARTESIAN_POINT ( 'NONE',  ( -1.035533905932738863, 61.50000000000000000, 48.54999999999999716 ) ) ;
#9774=SURFACE_SIDE_STYLE ('',( #9951 ) ) ;
#9785=CYLINDRICAL_SURFACE ( 'NONE', #3475, 2.500000000000002220 ) ;
#9802=ORIENTED_EDGE ( 'NONE', *, *, #14757, .T. ) ;
#9803=EDGE_CURVE ( 'NONE', #16441, #15290, #3497, .T. ) ;
#9805=LINE ( 'NONE', #10085, #8719 ) ;
#9807=CARTESIAN_POINT ( 'NONE',  ( 2.500000000000001776, 64.00000000000000000, 34.99999999999999289 ) ) ;
#9815=LINE ( 'NONE', #15810, #5371 ) ;
#9821=CARTESIAN_POINT ( 'NONE',  ( -2.066987300000001859, 64.85617417291294373, 48.70000000109247651 ) ) ;
#9828=ADVANCED_FACE ( 'NONE', ( #14472 ), #12987, .F. ) ;
#9833=CARTESIAN_POINT ( 'NONE',  ( -0.8561741729129465073, 61.93301270000000613, 45.90000000109247225 ) ) ;
#9837=LINE ( 'NONE', #14455, #16481 ) ;
#9846=CARTESIAN_POINT ( 'NONE',  ( -2.066987300000001859, 64.85617417291294373, 47.30000000109247082 ) ) ;
#9855=CARTESIAN_POINT ( 'NONE',  ( -2.500000000000001776, 64.00000000000000000, 47.59999999999999432 ) ) ;
#9856=CARTESIAN_POINT ( 'NONE',  ( -2.499999999999984013, 62.96446609406724804, 48.45000000000000284 ) ) ;
#9857=EDGE_CURVE ( 'NONE', #908, #17649, #17609, .T. ) ;
#9870=EDGE_CURVE ( 'NONE', #13549, #10345, #14134, .T. ) ;
#9885=AXIS2_PLACEMENT_3D ( 'NONE', #15531, #624, #2103 ) ;
#9896=VECTOR ( 'NONE', #3161, 1000.000000000000000 ) ;
#9898=CARTESIAN_POINT ( 'NONE',  ( -1.767766952966370209, 65.76776695296638309, 45.09999999999999432 ) ) ;
#9901=CARTESIAN_POINT ( 'NONE',  ( 41.00000000000000000, 52.00000000000000711, 30.00000000000000000 ) ) ;
#9905=CARTESIAN_POINT ( 'NONE',  ( -2.500000000000001776, 64.00000000000000000, 45.30000000218493739 ) ) ;
#9915=CARTESIAN_POINT ( 'NONE',  ( -1.461580736456473462, 62.53841926354353120, 48.05000000109247082 ) ) ;
#9918=FACE_BOUND ( 'NONE', #13490, .T. ) ;
#9924=CARTESIAN_POINT ( 'NONE',  ( 1.035533905932739751, 61.50000000000000000, 48.64999999999999858 ) ) ;
#9925=CARTESIAN_POINT ( 'NONE',  ( -0.8561741729129466183, 61.93301270000000613, 49.10000000109246088 ) ) ;
#9932=CARTESIAN_POINT ( 'NONE',  ( 1.461580736456473684, 65.46158073645646880, 46.85000000109246798 ) ) ;
#9935=EDGE_CURVE ( 'NONE', #7747, #2559, #1341, .T. ) ;
#9937=CARTESIAN_POINT ( 'NONE',  ( -1.461580736456473462, 62.53841926354353120, 48.25000000109246656 ) ) ;
#9940=CARTESIAN_POINT ( 'NONE',  ( 2.500000000000002220, 62.96446609406726225, 45.65000000218494591 ) ) ;
#9946=EDGE_CURVE ( 'NONE', #3632, #15274, #10244, .T. ) ;
#9949=ORIENTED_EDGE ( 'NONE', *, *, #6035, .F. ) ;
#9951=SURFACE_STYLE_FILL_AREA ( #1048 ) ;
#9954=ORIENTED_EDGE ( 'NONE', *, *, #15603, .F. ) ;
#9960=CARTESIAN_POINT ( 'NONE',  ( 0.000000000000000000, 47.00000000000000711, 30.00000000000000000 ) ) ;
#9972=CIRCLE ( 'NONE', #9354, 2.500000000000002220 ) ;
#9985=ADVANCED_FACE ( 'NONE', ( #13579 ), #2803, .F. ) ;
#9991=VECTOR ( 'NONE', #11329, 1000.000000000000000 ) ;
#10004=VECTOR ( 'NONE', #15780, 1000.000000000000000 ) ;
#10011=CARTESIAN_POINT ( 'NONE',  ( -1.461580736456473906, 65.46158073645646880, 47.05000000109247082 ) ) ;
#10014=VERTEX_POINT ( 'NONE', #11812 ) ;
#10023=CARTESIAN_POINT ( 'NONE',  ( -1.035533905932738863, 61.50000000000000000, 46.95000000000000995 ) ) ;
#10024=CARTESIAN_POINT ( 'NONE',  ( -2.500000000000003553, 62.96446609406726225, 49.24999999999997868 ) ) ;
#10026=CARTESIAN_POINT ( 'NONE',  ( -1.035533905932738863, 61.50000000000000000, 48.65000000218493881 ) ) ;
#10028=CARTESIAN_POINT ( 'NONE',  ( -2.500000000000001776, 64.00000000000000000, 48.39999999999999858 ) ) ;
#10034=CARTESIAN_POINT ( 'NONE',  ( -1.265664690411616068E-16, 66.06698730000000808, 44.55000000109247082 ) ) ;
#10040=CARTESIAN_POINT ( 'NONE',  ( 0.8561741729129460632, 66.06698729999999387, 48.70000000109247651 ) ) ;
#10060=LINE ( 'NONE', #2426, #16989 ) ;
#10063=ORIENTED_EDGE ( 'NONE', *, *, #4708, .F. ) ;
#10070=DIRECTION ( 'NONE',  ( -0.000000000000000000, -0.000000000000000000, -1.000000000000000000 ) ) ;
#10076=ORIENTED_EDGE ( 'NONE', *, *, #7601, .F. ) ;
#10085=CARTESIAN_POINT ( 'NONE',  ( -3.999999999999996447, 47.00000000000000711, 34.99999999999999289 ) ) ;
#10088=CARTESIAN_POINT ( 'NONE',  ( -2.500000000000001776, 64.00000000000000000, 47.59999999999999432 ) ) ;
#10096=CARTESIAN_POINT ( 'NONE',  ( -2.500000000000001776, 64.00000000000000000, 49.99999999999999289 ) ) ;
#10105=CARTESIAN_POINT ( 'NONE',  ( 0.8561741729129472844, 61.93301270000000613, 46.60000000109246088 ) ) ;
#10113=CARTESIAN_POINT ( 'NONE',  ( 1.035533905932738197, 66.50000000000000000, 45.05000000218493739 ) ) ;
#10116=CARTESIAN_POINT ( 'NONE',  ( -2.500000000000000888, 62.96446609406726935, 47.64999999999999858 ) ) ;
#10117=CARTESIAN_POINT ( 'NONE',  ( -1.461580736456473906, 65.46158073645646880, 49.65000000109246514 ) ) ;
#10130=CARTESIAN_POINT ( 'NONE',  ( -1.265664690411616068E-16, 66.06698730000000808, 47.15000000109247225 ) ) ;
#10133=LINE ( 'NONE', #12982, #9121 ) ;
#10139=CARTESIAN_POINT ( 'NONE',  ( 2.500000000000001776, 64.00000000000000000, 48.79999999999999716 ) ) ;
#10140=CARTESIAN_POINT ( 'NONE',  ( 4.592425496802577917E-16, 61.50000000000000000, 44.70000000218494307 ) ) ;
#10142=ORIENTED_EDGE ( 'NONE', *, *, #16772, .T. ) ;
#10144=ORIENTED_EDGE ( 'NONE', *, *, #9414, .F. ) ;
#10156=ORIENTED_EDGE ( 'NONE', *, *, #1505, .F. ) ;
#10160=CARTESIAN_POINT ( 'NONE',  ( -2.500000000000001776, 64.00000000000000000, 49.99999999999999289 ) ) ;
#10165=VECTOR ( 'NONE', #15926, 1000.000000000000000 ) ;
#10167=ORIENTED_EDGE ( 'NONE', *, *, #6725, .T. ) ;
#10179=ORIENTED_EDGE ( 'NONE', *, *, #756, .T. ) ;
#10185=AXIS2_PLACEMENT_3D ( 'NONE', #3181, #341, #16615 ) ;
#10193=CARTESIAN_POINT ( 'NONE',  ( -24.00000000000000000, 0.000000000000000000, -67.72004514666936359 ) ) ;
#10199=AXIS2_PLACEMENT_3D ( 'NONE', #1691, #7277, #5805 ) ;
#10201=ORIENTED_EDGE ( 'NONE', *, *, #14752, .F. ) ;
#10203=EDGE_CURVE ( 'NONE', #19297, #16534, #9134, .T. ) ;
#10206=CARTESIAN_POINT ( 'NONE',  ( 2.066987300000002303, 63.14382582708705627, 45.90000000109247225 ) ) ;
#10215=FACE_BOUND ( 'NONE', #19289, .T. ) ;
#10219=EDGE_CURVE ( 'NONE', #18580, #15589, #9815, .T. ) ;
#10220=CARTESIAN_POINT ( 'NONE',  ( -1.767766952966369765, 62.23223304703363112, 46.09999999999999432 ) ) ;
#10221=CARTESIAN_POINT ( 'NONE',  ( -2.066987300000001415, 64.00000000000000000, 45.75000000109247367 ) ) ;
#10222=ADVANCED_FACE ( 'NONE', ( #18858 ), #18577, .F. ) ;
#10235=CARTESIAN_POINT ( 'NONE',  ( -2.066987300000001415, 64.00000000000000000, 47.35000000109246798 ) ) ;
#10244=LINE ( 'NONE', #4284, #13488 ) ;
#10254=LINE ( 'NONE', #1354, #2869 ) ;
#10261=ORIENTED_EDGE ( 'NONE', *, *, #3875, .F. ) ;
#10267=DIRECTION ( 'NONE',  ( -0.000000000000000000, -1.000000000000000000, -0.000000000000000000 ) ) ;
#10275=ORIENTED_EDGE ( 'NONE', *, *, #4708, .T. ) ;
#10282=CARTESIAN_POINT ( 'NONE',  ( -1.767766952966370209, 65.76776695296638309, 44.40000000218493881 ) ) ;
#10284=CARTESIAN_POINT ( 'NONE',  ( 0.000000000000000000, 47.00000000000000711, 30.00000000000000000 ) ) ;
#10293=CARTESIAN_POINT ( 'NONE',  ( -2.500000000000001776, 64.00000000000000000, 34.99999999999999289 ) ) ;
#10295=AXIS2_PLACEMENT_3D ( 'NONE', #17975, #15034, #4456 ) ;
#10296=FACE_OUTER_BOUND ( 'NONE', #5676, .T. ) ;
#10308=ORIENTED_EDGE ( 'NONE', *, *, #15118, .F. ) ;
#10312=CARTESIAN_POINT ( 'NONE',  ( -1.767766952966370209, 65.76776695296638309, 45.20000000218494307 ) ) ;
#10315=CARTESIAN_POINT ( 'NONE',  ( -1.530808498934192803E-16, 66.50000000000000000, 46.59999999999999432 ) ) ;
#10316=CARTESIAN_POINT ( 'NONE',  ( 1.461580736456473684, 65.46158073645646880, 47.05000000109247082 ) ) ;
#10328=CARTESIAN_POINT ( 'NONE',  ( -1.530808498934192803E-16, 66.50000000000000000, 48.30000000218494449 ) ) ;
#10332=CARTESIAN_POINT ( 'NONE',  ( -2.066987300000001415, 64.00000000000000000, 45.75000000109247367 ) ) ;
#10345=VERTEX_POINT ( 'NONE', #10776 ) ;
#10352=ORIENTED_EDGE ( 'NONE', *, *, #11635, .F. ) ;
#10359=FACE_OUTER_BOUND ( 'NONE', #14983, .T. ) ;
#10370=DIRECTION ( 'NONE',  ( 0.000000000000000000, 0.000000000000000000, 1.000000000000000000 ) ) ;
#10381=ORIENTED_EDGE ( 'NONE', *, *, #9440, .T. ) ;
#10386=VERTEX_POINT ( 'NONE', #9605 ) ;
#10388=ORIENTED_EDGE ( 'NONE', *, *, #11381, .T. ) ;
#10397=CARTESIAN_POINT ( 'NONE',  ( 2.500000000000006661, 65.03553390593272354, 48.04999999999999716 ) ) ;
#10403=CARTESIAN_POINT ( 'NONE',  ( -2.066987300000001859, 64.85617417291294373, 44.70000000109248361 ) ) ;
#10411=CARTESIAN_POINT ( 'NONE',  ( 1.035533905932739751, 61.50000000000000000, 45.44999999999999574 ) ) ;
#10412=DIRECTION ( 'NONE',  ( 0.000000000000000000, 1.000000000000000000, -0.000000000000000000 ) ) ;
#10414=CARTESIAN_POINT ( 'NONE',  ( -1.461580736456473906, 65.46158073645646880, 45.65000000109247225 ) ) ;
#10419=ADVANCED_FACE ( 'NONE', ( #14122 ), #12450, .F. ) ;
#10427=CARTESIAN_POINT ( 'NONE',  ( 1.461580736456473906, 62.53841926354353120, 45.25000000109247367 ) ) ;
#10447=ORIENTED_EDGE ( 'NONE', *, *, #57, .F. ) ;
#10451=CARTESIAN_POINT ( 'NONE',  ( -4.000000000000001776, 67.00000000000000000, 34.99999999999999289 ) ) ;
#10453=CARTESIAN_POINT ( 'NONE',  ( -2.066987300000001415, 64.00000000000000000, 49.55000000109247082 ) ) ;
#10468=ORIENTED_EDGE ( 'NONE', *, *, #18776, .T. ) ;
#10483=CARTESIAN_POINT ( 'NONE',  ( -1.035533905932738641, 66.50000000000000000, 47.55000000218494449 ) ) ;
#10488=CARTESIAN_POINT ( 'NONE',  ( -32.50000000000000000, 47.00000000000000711, 15.00000000000000000 ) ) ;
#10502=CARTESIAN_POINT ( 'NONE',  ( -0.8561741729129465073, 61.93301270000000613, 45.70000000109248361 ) ) ;
#10512=CARTESIAN_POINT ( 'NONE',  ( 2.066987300000001859, 63.14382582708704916, 46.10000000109246798 ) ) ;
#10528=CARTESIAN_POINT ( 'NONE',  ( -1.265664690411616068E-16, 66.06698730000000808, 45.55000000109246372 ) ) ;
#10539=ADVANCED_FACE ( 'NONE', ( #12919 ), #17162, .T. ) ;
#10541=COLOUR_RGB ( '', 0.66274510, 0.83137255, 0.94901961) ;
#10548=CARTESIAN_POINT ( 'NONE',  ( -15.00000000000000000, 35.00000000000000000, 0.000000000000000000 ) ) ;
#10554=CARTESIAN_POINT ( 'NONE',  ( 0.8561741729129472844, 61.93301270000000613, 49.00000000109246656 ) ) ;
#10556=ORIENTED_EDGE ( 'NONE', *, *, #12722, .F. ) ;
#10567=VERTEX_POINT ( 'NONE', #18821 ) ;
#10586=CARTESIAN_POINT ( 'NONE',  ( 2.500000000000001776, 64.00000000000000000, 46.39999999999999858 ) ) ;
#10590=CARTESIAN_POINT ( 'NONE',  ( -15.00000000000000000, 35.00000000000000000, 33.99999999999999289 ) ) ;
#10595=DIRECTION ( 'NONE',  ( -0.000000000000000000, -0.000000000000000000, -1.000000000000000000 ) ) ;
#10596=ORIENTED_EDGE ( 'NONE', *, *, #3850, .F. ) ;
#10610=CARTESIAN_POINT ( 'NONE',  ( 2.066987300000001415, 64.00000000000000000, 46.95000000109246940 ) ) ;
#10616=EDGE_CURVE ( 'NONE', #18125, #17611, #13673, .T. ) ;
#10621=CARTESIAN_POINT ( 'NONE',  ( 1.767766952966370653, 62.23223304703363112, 48.80000000218494449 ) ) ;
#10629=CARTESIAN_POINT ( 'NONE',  ( 0.8561741729129472844, 61.93301270000000613, 49.20000000109247651 ) ) ;
#10635=DIRECTION ( 'NONE',  ( -1.000000000000000000, 0.000000000000000000, 0.000000000000000000 ) ) ;
#10639=ORIENTED_EDGE ( 'NONE', *, *, #10695, .T. ) ;
#10647=CARTESIAN_POINT ( 'NONE',  ( -15.00000000000000000, 0.000000000000000000, 33.99999999999999289 ) ) ;
#10650=CARTESIAN_POINT ( 'NONE',  ( 3.796994071234847710E-16, 61.93301269999999903, 48.95000000109246940 ) ) ;
#10659=CARTESIAN_POINT ( 'NONE',  ( 0.000000000000000000, 52.00000000000000711, -50.00000000000000000 ) ) ;
#10678=CARTESIAN_POINT ( 'NONE',  ( -0.8561741729129461742, 66.06698730000000808, 47.80000000109247082 ) ) ;
#10691=DIRECTION ( 'NONE',  ( 0.000000000000000000, 0.000000000000000000, 1.000000000000000000 ) ) ;
#10695=EDGE_CURVE ( 'NONE', #18430, #18471, #7491, .T. ) ;
#10696=CARTESIAN_POINT ( 'NONE',  ( 24.00000000000000000, 47.00000000000000711, -50.00000000000000000 ) ) ;
#10697=EDGE_LOOP ( 'NONE', ( #18609, #10556, #7237, #9694 ) ) ;
#10703=APPLICATION_CONTEXT ( 'automotive_design' ) ;
#10717=CARTESIAN_POINT ( 'NONE',  ( -32.50000000000000000, 47.00000000000000711, -35.00000000000000000 ) ) ;
#10720=ORIENTED_EDGE ( 'NONE', *, *, #3941, .T. ) ;
#10721=ADVANCED_FACE ( 'NONE', ( #354 ), #6341, .T. ) ;
#10724=CARTESIAN_POINT ( 'NONE',  ( -1.530808498934192803E-16, 66.50000000000000000, 45.90000000218494591 ) ) ;
#10731=CARTESIAN_POINT ( 'NONE',  ( -2.500000000000006661, 65.03553390593272354, 45.94999999999999574 ) ) ;
#10733=CARTESIAN_POINT ( 'NONE',  ( -1.265664690411616068E-16, 66.06698730000000808, 46.35000000109246798 ) ) ;
#10768=CARTESIAN_POINT ( 'NONE',  ( 2.066987300000001859, 63.14382582708704916, 47.50000000109246656 ) ) ;
#10776=CARTESIAN_POINT ( 'NONE',  ( -32.50000000000000000, 52.00000000000000711, -37.50000000000000711 ) ) ;
#10785=ADVANCED_FACE ( 'NONE', ( #17599 ), #14269, .F. ) ;
#10806=PLANE ( 'NONE',  #17688 ) ;
#10809=DIRECTION ( 'NONE',  ( 0.000000000000000000, 0.000000000000000000, 1.000000000000000000 ) ) ;
#10818=CARTESIAN_POINT ( 'NONE',  ( 4.592425496802577917E-16, 61.50000000000000000, 45.50000000218494733 ) ) ;
#10820=ADVANCED_FACE ( 'NONE', ( #13175 ), #3791, .F. ) ;
#10832=CARTESIAN_POINT ( 'NONE',  ( 3.796994071234847710E-16, 61.93301269999999903, 47.55000000109247082 ) ) ;
#10844=ORIENTED_EDGE ( 'NONE', *, *, #2088, .F. ) ;
#10845=ADVANCED_FACE ( 'NONE', ( #14359 ), #8297, .F. ) ;
#10850=CARTESIAN_POINT ( 'NONE',  ( 1.461580736456473906, 62.53841926354353120, 45.05000000109246372 ) ) ;
#10852=ORIENTED_EDGE ( 'NONE', *, *, #10616, .F. ) ;
#10853=ORIENTED_EDGE ( 'NONE', *, *, #16339, .F. ) ;
#10872=( BOUNDED_CURVE ( )  B_SPLINE_CURVE ( 2, ( #8450, #5603, #8359, #4033, #16001, #2563, #19135, #14518, #1089 ),
 .UNSPECIFIED., .F., .F. ) 
 B_SPLINE_CURVE_WITH_KNOTS ( ( 3, 2, 2, 2, 3 ),
 ( 0.2142857142857140795, 0.2321428571428570675, 0.2500000000000000000, 0.2678571428571429602, 0.2857142857142859205 ),
 .UNSPECIFIED. ) 
 CURVE ( )  GEOMETRIC_REPRESENTATION_ITEM ( )  RATIONAL_B_SPLINE_CURVE ( ( 1.000000000000000888, 0.9238795325112859613, 1.000000000000000000, 0.9238795325112867385, 1.000000000000000000, 0.9238795325112867385, 1.000000000000000000, 0.9238795325112857393, 1.000000000000000888 ) ) 
 REPRESENTATION_ITEM ( '' )  );
#10887=CARTESIAN_POINT ( 'NONE',  ( 1.767766952966369987, 65.76776695296638309, 49.00000000218494023 ) ) ;
#10891=ORIENTED_EDGE ( 'NONE', *, *, #4238, .F. ) ;
#10901=CARTESIAN_POINT ( 'NONE',  ( -4.000000000000001776, 67.00000000000000000, 34.99999999999999289 ) ) ;
#10907=CARTESIAN_POINT ( 'NONE',  ( 0.8561741729129471734, 61.93301270000000613, 45.20000000109248361 ) ) ;
#10915=CARTESIAN_POINT ( 'NONE',  ( 2.500000000000001776, 65.03553390593273775, 45.75000000218494023 ) ) ;
#10916=ADVANCED_FACE ( 'NONE', ( #2788 ), #117, .T. ) ;
#10925=CARTESIAN_POINT ( 'NONE',  ( 0.8561741729129472844, 61.93301270000000613, 46.80000000109246372 ) ) ;
#10926=CARTESIAN_POINT ( 'NONE',  ( 1.767766952966370653, 62.23223304703363112, 49.49999999999999289 ) ) ;
#10933=ORIENTED_EDGE ( 'NONE', *, *, #851, .T. ) ;
#10944=CARTESIAN_POINT ( 'NONE',  ( 3.796994071234847710E-16, 61.93301269999999903, 45.75000000109247367 ) ) ;
#10967=CARTESIAN_POINT ( 'NONE',  ( 1.461580736456473684, 65.46158073645646880, 47.65000000109247225 ) ) ;
#10970=B_SPLINE_CURVE_WITH_KNOTS ( 'NONE', 1,
 ( #6162, #12219 ),
 .UNSPECIFIED., .F., .F.,
 ( 2, 2 ),
 ( 0.000000000000000000, 1.000000000000000000 ),
 .UNSPECIFIED. ) ;
#11000=DIRECTION ( 'NONE',  ( 1.000000000000000000, -0.000000000000000000, 0.000000000000000000 ) ) ;
#11012=ORIENTED_EDGE ( 'NONE', *, *, #2784, .T. ) ;
#11015=CARTESIAN_POINT ( 'NONE',  ( -2.500000000000001776, 64.00000000000000000, 45.30000000218493739 ) ) ;
#11023=CARTESIAN_POINT ( 'NONE',  ( -1.461580736456473462, 62.53841926354353120, 47.45000000109246230 ) ) ;
#11039=EDGE_CURVE ( 'NONE', #4427, #3539, #6574, .T. ) ;
#11041=CARTESIAN_POINT ( 'NONE',  ( -2.066987300000001415, 63.14382582708705627, 47.20000000109248361 ) ) ;
#11042=DIRECTION ( 'NONE',  ( 0.000000000000000000, 1.000000000000000000, 0.000000000000000000 ) ) ;
#11048=CARTESIAN_POINT ( 'NONE',  ( -41.00000000000000000, 52.00000000000000711, 18.00000000000000000 ) ) ;
#11049=EDGE_CURVE ( 'NONE', #3710, #10567, #14147, .T. ) ;
#11058=ORIENTED_EDGE ( 'NONE', *, *, #1942, .F. ) ;
#11067=DIRECTION ( 'NONE',  ( -0.000000000000000000, 1.000000000000000000, 0.000000000000000000 ) ) ;
#11086=EDGE_LOOP ( 'NONE', ( #2372, #11583, #5663, #1968 ) ) ;
#11102=DIRECTION ( 'NONE',  ( 0.000000000000000000, 1.000000000000000000, 0.000000000000000000 ) ) ;
#11109=ADVANCED_FACE ( 'NONE', ( #14294 ), #2250, .T. ) ;
#11110=CARTESIAN_POINT ( 'NONE',  ( -2.500000000000000888, 62.96446609406726935, 45.35000000218493454 ) ) ;
#11114=FACE_OUTER_BOUND ( 'NONE', #15315, .T. ) ;
#11118=CARTESIAN_POINT ( 'NONE',  ( -1.767766952966370209, 65.76776695296638309, 49.89999999999999147 ) ) ;
#11121=LINE ( 'NONE', #10096, #9750 ) ;
#11122=AXIS2_PLACEMENT_3D ( 'NONE', #4973, #2021, #12111 ) ;
#11128=CARTESIAN_POINT ( 'NONE',  ( -2.066987300000000971, 63.14382582708704916, 44.80000000109247082 ) ) ;
#11132=AXIS2_PLACEMENT_3D ( 'NONE', #1190, #3948, #17664 ) ;
#11134=CARTESIAN_POINT ( 'NONE',  ( 2.066987300000001859, 64.85617417291294373, 46.00000000109246656 ) ) ;
#11156=CARTESIAN_POINT ( 'NONE',  ( 32.50000000000000000, 52.00000000000000711, -37.50000000000000711 ) ) ;
#11172=ORIENTED_EDGE ( 'NONE', *, *, #2682, .F. ) ;
#11181=CARTESIAN_POINT ( 'NONE',  ( -2.500000000000001776, 65.03553390593273775, 45.14999999999999858 ) ) ;
#11192=CARTESIAN_POINT ( 'NONE',  ( 32.50000000000000000, 47.00000000000000711, -35.00000000000000000 ) ) ;
#11198=CARTESIAN_POINT ( 'NONE',  ( -1.265664690411616068E-16, 66.06698730000000808, 49.35000000109246798 ) ) ;
#11206=CARTESIAN_POINT ( 'NONE',  ( -1.767766952966370209, 65.76776695296638309, 49.09999999999999432 ) ) ;
#11210=CARTESIAN_POINT ( 'NONE',  ( 0.000000000000000000, 52.00000000000000711, 30.00000000000000000 ) ) ;
#11214=CARTESIAN_POINT ( 'NONE',  ( 2.066987300000001415, 64.00000000000000000, 45.95000000109246940 ) ) ;
#11216=EDGE_CURVE ( 'NONE', #292, #3881, #10060, .T. ) ;
#11219=VECTOR ( 'NONE', #7240, 1000.000000000000000 ) ;
#11220=CARTESIAN_POINT ( 'NONE',  ( -1.461580736456473906, 65.46158073645646880, 45.45000000109246940 ) ) ;
#11226=DIRECTION ( 'NONE',  ( 0.000000000000000000, 0.000000000000000000, 1.000000000000000000 ) ) ;
#11245=ORIENTED_EDGE ( 'NONE', *, *, #3755, .T. ) ;
#11259=( BOUNDED_CURVE ( )  B_SPLINE_CURVE ( 2, ( #3781, #8663, #2686, #11495, #3869, #10026, #12969, #17483, #925 ),
 .UNSPECIFIED., .F., .F. ) 
 B_SPLINE_CURVE_WITH_KNOTS ( ( 3, 2, 2, 2, 3 ),
 ( 0.07142857142857156338, 0.08928571428571438484, 0.1071428571428571924, 0.1250000000000000000, 0.1428571428571428215 ),
 .UNSPECIFIED. ) 
 CURVE ( )  GEOMETRIC_REPRESENTATION_ITEM ( )  RATIONAL_B_SPLINE_CURVE ( ( 0.9999999999999994449, 0.9238795325112872936, 1.000000000000000000, 0.9238795325112867385, 1.000000000000000000, 0.9238795325112867385, 1.000000000000000000, 0.9238795325112868495, 0.9999999999999998890 ) ) 
 REPRESENTATION_ITEM ( '' )  );
#11273=CARTESIAN_POINT ( 'NONE',  ( 1.035533905932738197, 66.50000000000000000, 45.75000000000000000 ) ) ;
#11275=CARTESIAN_POINT ( 'NONE',  ( -3.999999999999996447, 47.00000000000000711, 34.99999999999999289 ) ) ;
#11278=CARTESIAN_POINT ( 'NONE',  ( -2.500000000000001776, 64.00000000000000000, 46.90000000218494591 ) ) ;
#11287=EDGE_CURVE ( 'NONE', #3899, #17145, #10254, .T. ) ;
#11290=DIRECTION ( 'NONE',  ( 0.000000000000000000, 0.000000000000000000, 1.000000000000000000 ) ) ;
#11297=CARTESIAN_POINT ( 'NONE',  ( 1.461580736456473906, 62.53841926354353120, 46.65000000109247225 ) ) ;
#11300=CARTESIAN_POINT ( 'NONE',  ( 2.500000000000001776, 64.00000000000000000, 46.50000000218494733 ) ) ;
#11309=CARTESIAN_POINT ( 'NONE',  ( 2.500000000000002220, 62.96446609406726935, 49.54999999999999716 ) ) ;
#11310=CARTESIAN_POINT ( 'NONE',  ( 2.066987300000001415, 64.85617417291294373, 49.40000000109246514 ) ) ;
#11322=CARTESIAN_POINT ( 'NONE',  ( -2.066987300000001415, 64.00000000000000000, 48.15000000109247225 ) ) ;
#11329=DIRECTION ( 'NONE',  ( -0.000000000000000000, -0.000000000000000000, -1.000000000000000000 ) ) ;
#11334=EDGE_LOOP ( 'NONE', ( #31, #1456, #8054, #18151 ) ) ;
#11347=CARTESIAN_POINT ( 'NONE',  ( -2.500000000000001776, 64.00000000000000000, 46.10000000218494165 ) ) ;
#11356=CARTESIAN_POINT ( 'NONE',  ( -10.00000000000000000, 49.99999999999997158, -4.956352788505161414E-14 ) ) ;
#11362=ORIENTED_EDGE ( 'NONE', *, *, #2682, .T. ) ;
#11364=CARTESIAN_POINT ( 'NONE',  ( -1.035533905932738641, 66.50000000000000000, 45.84999999999998721 ) ) ;
#11375=DIRECTION ( 'NONE',  ( 0.000000000000000000, 0.000000000000000000, 1.000000000000000000 ) ) ;
#11381=EDGE_CURVE ( 'NONE', #19221, #15669, #3198, .T. ) ;
#11386=CARTESIAN_POINT ( 'NONE',  ( 1.461580736456473906, 62.53841926354353120, 48.25000000109246656 ) ) ;
#11395=CARTESIAN_POINT ( 'NONE',  ( 41.00000000000000000, 52.00000000000000711, -50.00000000000000000 ) ) ;
#11396=CARTESIAN_POINT ( 'NONE',  ( -2.500000000000000888, 62.96446609406726935, 49.24999999999999289 ) ) ;
#11397=CARTESIAN_POINT ( 'NONE',  ( -1.265664690411616068E-16, 66.06698730000000808, 48.75000000109246656 ) ) ;
#11404=ADVANCED_FACE ( 'NONE', ( #10359 ), #4770, .T. ) ;
#11405=CARTESIAN_POINT ( 'NONE',  ( 0.8561741729129460632, 66.06698730000000808, 46.90000000109247225 ) ) ;
#11408=DIRECTION ( 'NONE',  ( 1.000000000000000000, 2.602085213965211135E-16, -0.000000000000000000 ) ) ;
#11411=CARTESIAN_POINT ( 'NONE',  ( -1.265664690411616068E-16, 66.06698730000000808, 44.55000000109247082 ) ) ;
#11414=CARTESIAN_POINT ( 'NONE',  ( 14.99999999999998579, 47.00000000000000711, 26.99999999999997158 ) ) ;
#11415=CARTESIAN_POINT ( 'NONE',  ( 4.592425496802577917E-16, 61.50000000000000000, 45.50000000218494733 ) ) ;
#11421=DIRECTION ( 'NONE',  ( -0.000000000000000000, -1.000000000000000000, -0.000000000000000000 ) ) ;
#11428=EDGE_LOOP ( 'NONE', ( #8832, #5979, #13447, #10352, #16941, #7829, #13408, #13206, #10596, #17155 ) ) ;
#11430=ORIENTED_EDGE ( 'NONE', *, *, #11659, .T. ) ;
#11435=DIRECTION ( 'NONE',  ( -0.000000000000000000, -0.000000000000000000, -1.000000000000000000 ) ) ;
#11442=ORIENTED_EDGE ( 'NONE', *, *, #3875, .T. ) ;
#11453=VERTEX_POINT ( 'NONE', #4776 ) ;
#11457=ORIENTED_EDGE ( 'NONE', *, *, #12109, .T. ) ;
#11460=CIRCLE ( 'NONE', #12415, 2.500000000000002220 ) ;
#11462=ORIENTED_EDGE ( 'NONE', *, *, #11635, .T. ) ;
#11467=CARTESIAN_POINT ( 'NONE',  ( 14.99999999999998579, 52.00000000000000711, 20.99999999999997513 ) ) ;
#11470=LINE ( 'NONE', #17762, #979 ) ;
#11477=CARTESIAN_POINT ( 'NONE',  ( -2.500000000000001776, 64.00000000000000000, 46.00000000000000000 ) ) ;
#11481=CARTESIAN_POINT ( 'NONE',  ( 1.461580736456473906, 62.53841926354353120, 49.05000000109247082 ) ) ;
#11486=FACE_BOUND ( 'NONE', #1584, .T. ) ;
#11489=CARTESIAN_POINT ( 'NONE',  ( 41.00000000000000000, 47.00000000000000711, 18.00000000000000000 ) ) ;
#11492=CARTESIAN_POINT ( 'NONE',  ( -0.8561741729129461742, 66.06698729999999387, 44.80000000109246372 ) ) ;
#11493=CARTESIAN_POINT ( 'NONE',  ( 2.066987300000001415, 64.00000000000000000, 48.55000000109247082 ) ) ;
#11495=CARTESIAN_POINT ( 'NONE',  ( 1.035533905932739751, 61.50000000000000000, 48.75000000218494023 ) ) ;
#11498=ORIENTED_EDGE ( 'NONE', *, *, #4238, .T. ) ;
#11500=CARTESIAN_POINT ( 'NONE',  ( -0.8561741729129466183, 61.93301270000000613, 46.50000000109247367 ) ) ;
#11504=CARTESIAN_POINT ( 'NONE',  ( -1.265664690411616068E-16, 66.06698730000000808, 47.95000000109246940 ) ) ;
#11512=DIRECTION ( 'NONE',  ( 0.000000000000000000, 0.000000000000000000, 1.000000000000000000 ) ) ;
#11515=CARTESIAN_POINT ( 'NONE',  ( -2.499999999999992006, 62.96446609406726225, 44.55000000218494449 ) ) ;
#11525=VECTOR ( 'NONE', #19054, 1000.000000000000000 ) ;
#11539=EDGE_CURVE ( 'NONE', #11453, #14781, #17203, .T. ) ;
#11554=CARTESIAN_POINT ( 'NONE',  ( -1.530808498934192803E-16, 66.50000000000000000, 45.00000000000000000 ) ) ;
#11559=ORIENTED_EDGE ( 'NONE', *, *, #420, .T. ) ;
#11563=DIRECTION ( 'NONE',  ( 0.000000000000000000, 1.000000000000000000, 0.000000000000000000 ) ) ;
#11580=CARTESIAN_POINT ( 'NONE',  ( 2.066987300000001859, 64.85617417291294373, 49.20000000109247651 ) ) ;
#11583=ORIENTED_EDGE ( 'NONE', *, *, #15603, .T. ) ;
#11585=CARTESIAN_POINT ( 'NONE',  ( 2.500000000000004441, 62.96446609406726225, 46.45000000218494307 ) ) ;
#11589=LINE ( 'NONE', #4163, #6840 ) ;
#11591=CARTESIAN_POINT ( 'NONE',  ( 4.592425496802577917E-16, 61.50000000000000000, 46.99999999999999289 ) ) ;
#11599=CIRCLE ( 'NONE', #7877, 2.500000000000001776 ) ;
#11605=CARTESIAN_POINT ( 'NONE',  ( 1.461580736456473684, 65.46158073645646880, 48.65000000109247225 ) ) ;
#11615=CARTESIAN_POINT ( 'NONE',  ( -1.035533905932738863, 61.50000000000000000, 47.74999999999999289 ) ) ;
#11618=ADVANCED_FACE ( 'NONE', ( #5151 ), #9643, .T. ) ;
#11625=CARTESIAN_POINT ( 'NONE',  ( -2.500000000000001776, 64.00000000000000000, 49.19999999999999574 ) ) ;
#11635=EDGE_CURVE ( 'NONE', #3717, #4896, #18584, .T. ) ;
#11640=FACE_OUTER_BOUND ( 'NONE', #6844, .T. ) ;
#11647=ORIENTED_EDGE ( 'NONE', *, *, #3941, .F. ) ;
#11657=CARTESIAN_POINT ( 'NONE',  ( -1.530808498934192803E-16, 66.50000000000000000, 45.00000000000000000 ) ) ;
#11659=EDGE_CURVE ( 'NONE', #11681, #4215, #6754, .T. ) ;
#11661=CARTESIAN_POINT ( 'NONE',  ( -2.500000000000001776, 64.00000000000000000, 44.50000000218494733 ) ) ;
#11666=ADVANCED_FACE ( 'NONE', ( #19154, #3861, #17474, #9918, #5724, #11486, #15914 ), #8466, .T. ) ;
#11669=LINE ( 'NONE', #13238, #8813 ) ;
#11681=VERTEX_POINT ( 'NONE', #11300 ) ;
#11685=CARTESIAN_POINT ( 'NONE',  ( -1.035533905932738641, 66.50000000000000000, 45.15000000218493881 ) ) ;
#11690=CARTESIAN_POINT ( 'NONE',  ( -1.035533905932738863, 61.50000000000000000, 46.14999999999999858 ) ) ;
#11691=CARTESIAN_POINT ( 'NONE',  ( -2.066987300000000971, 63.14382582708704916, 46.60000000109246798 ) ) ;
#11696=ORIENTED_EDGE ( 'NONE', *, *, #4730, .F. ) ;
#11700=CARTESIAN_POINT ( 'NONE',  ( -2.500000000000001776, 65.03553390593273775, 48.45000000218495018 ) ) ;
#11702=CARTESIAN_POINT ( 'NONE',  ( 1.461580736456473684, 65.46158073645646880, 49.45000000109246940 ) ) ;
#11709=FACE_BOUND ( 'NONE', #2834, .T. ) ;
#11718=DIRECTION ( 'NONE',  ( 0.000000000000000000, 0.000000000000000000, 1.000000000000000000 ) ) ;
#11731=CARTESIAN_POINT ( 'NONE',  ( 3.999999999999998224, 67.00000000000000000, 34.99999999999999289 ) ) ;
#11737=CARTESIAN_POINT ( 'NONE',  ( -1.035533905932738863, 61.50000000000000000, 47.05000000218494449 ) ) ;
#11759=EDGE_LOOP ( 'NONE', ( #6052, #6664, #13326, #7265 ) ) ;
#11773=FACE_OUTER_BOUND ( 'NONE', #16775, .T. ) ;
#11791=CARTESIAN_POINT ( 'NONE',  ( -1.767766952966369765, 62.23223304703363112, 46.89999999999999858 ) ) ;
#11792=CARTESIAN_POINT ( 'NONE',  ( -2.066987300000001415, 64.85617417291294373, 46.50000000109246656 ) ) ;
#11801=CARTESIAN_POINT ( 'NONE',  ( 4.592425496802577917E-16, 61.50000000000000000, 48.70000000218494307 ) ) ;
#11812=CARTESIAN_POINT ( 'NONE',  ( 2.500000000000001776, 64.00000000000000000, 44.90000000218493881 ) ) ;
#11818=DIRECTION ( 'NONE',  ( 0.000000000000000000, -1.000000000000000000, 0.000000000000000000 ) ) ;
#11819=ORIENTED_EDGE ( 'NONE', *, *, #11539, .F. ) ;
#11848=PLANE ( 'NONE',  #13765 ) ;
#11851=VECTOR ( 'NONE', #10070, 1000.000000000000000 ) ;
#11856=DIRECTION ( 'NONE',  ( 0.000000000000000000, 0.000000000000000000, 1.000000000000000000 ) ) ;
#11876=CARTESIAN_POINT ( 'NONE',  ( -1.461580736456473906, 65.46158073645646880, 45.45000000109246940 ) ) ;
#11887=CARTESIAN_POINT ( 'NONE',  ( 2.500000000000001776, 64.00000000000000000, 45.59999999999999432 ) ) ;
#11891=CARTESIAN_POINT ( 'NONE',  ( -1.461580736456473462, 62.53841926354353120, 47.45000000109246230 ) ) ;
#11893=DIRECTION ( 'NONE',  ( 0.000000000000000000, 0.000000000000000000, 1.000000000000000000 ) ) ;
#11899=VECTOR ( 'NONE', #16779, 1000.000000000000000 ) ;
#11913=ADVANCED_FACE ( 'NONE', ( #1609 ), #3170, .T. ) ;
#11919=DIRECTION ( 'NONE',  ( 0.000000000000000000, -0.000000000000000000, -1.000000000000000000 ) ) ;
#11925=CARTESIAN_POINT ( 'NONE',  ( 0.000000000000000000, 0.000000000000000000, 30.00000000000000000 ) ) ;
#11950=ORIENTED_EDGE ( 'NONE', *, *, #1001, .T. ) ;
#11958=DIRECTION ( 'NONE',  ( 0.000000000000000000, 0.000000000000000000, 1.000000000000000000 ) ) ;
#11972=CARTESIAN_POINT ( 'NONE',  ( 0.000000000000000000, 64.00000000000000000, 49.99999999999999289 ) ) ;
#11987=CARTESIAN_POINT ( 'NONE',  ( 1.461580736456473684, 65.46158073645646880, 46.25000000109246656 ) ) ;
#11992=ORIENTED_EDGE ( 'NONE', *, *, #6786, .F. ) ;
#11995=CARTESIAN_POINT ( 'NONE',  ( -1.035533905932738863, 61.50000000000000000, 48.65000000218493881 ) ) ;
#12005=SHAPE_REPRESENTATION ( 'Spring-Loaded Carriage Elevator Arm', ( #1791 ), #13038 ) ;
#12021=ORIENTED_EDGE ( 'NONE', *, *, #18128, .F. ) ;
#12035=CARTESIAN_POINT ( 'NONE',  ( -10.00000000000000000, -0.000000000000000000, 37.00000000000000000 ) ) ;
#12037=EDGE_CURVE ( 'NONE', #18125, #8404, #4756, .T. ) ;
#12045=VERTEX_POINT ( 'NONE', #3616 ) ;
#12048=VECTOR ( 'NONE', #3659, 1000.000000000000000 ) ;
#12055=CARTESIAN_POINT ( 'NONE',  ( 2.500000000000001776, 64.00000000000000000, 47.30000000218494449 ) ) ;
#12075=CARTESIAN_POINT ( 'NONE',  ( -1.265664690411616068E-16, 66.06698730000000808, 44.55000000109247082 ) ) ;
#12077=DIRECTION ( 'NONE',  ( -1.000000000000000000, 0.000000000000000000, 0.000000000000000000 ) ) ;
#12079=DIRECTION ( 'NONE',  ( -0.000000000000000000, -0.000000000000000000, -1.000000000000000000 ) ) ;
#12080=EDGE_LOOP ( 'NONE', ( #18715, #18108, #14313, #13800 ) ) ;
#12081=FACE_OUTER_BOUND ( 'NONE', #11759, .T. ) ;
#12085=CARTESIAN_POINT ( 'NONE',  ( 1.461580736456473906, 62.53841926354353120, 48.45000000109246940 ) ) ;
#12089=LINE ( 'NONE', #1808, #4263 ) ;
#12098=CARTESIAN_POINT ( 'NONE',  ( -0.8561741729129461742, 66.06698729999999387, 45.60000000109246088 ) ) ;
#12103=CARTESIAN_POINT ( 'NONE',  ( 0.000000000000000000, 64.00000000000000000, 49.99999999999999289 ) ) ;
#12104=CARTESIAN_POINT ( 'NONE',  ( -2.066987300000001859, 64.85617417291294373, 46.50000000109246656 ) ) ;
#12109=EDGE_CURVE ( 'NONE', #14374, #11453, #13852, .T. ) ;
#12110=EDGE_CURVE ( 'NONE', #17649, #3686, #12467, .T. ) ;
#12111=DIRECTION ( 'NONE',  ( 0.000000000000000000, 0.000000000000000000, 1.000000000000000000 ) ) ;
#12112=( GEOMETRIC_REPRESENTATION_CONTEXT ( 3 ) GLOBAL_UNCERTAINTY_ASSIGNED_CONTEXT ( ( #439 ) ) GLOBAL_UNIT_ASSIGNED_CONTEXT ( ( #14477, #7025, #5561 ) ) REPRESENTATION_CONTEXT ( 'NONE', 'WORKASPACE' ) );
#12128=( BOUNDED_CURVE ( )  B_SPLINE_CURVE ( 2, ( #213, #3248, #16685, #1976, #15113, #6293, #12156, #4828, #10586 ),
 .UNSPECIFIED., .F., .F. ) 
 B_SPLINE_CURVE_WITH_KNOTS ( ( 3, 2, 2, 2, 3 ),
 ( 0.5714285714285713969, 0.5892857142857143016, 0.6071428571428569843, 0.6249999999999998890, 0.6428571428571427937 ),
 .UNSPECIFIED. ) 
 CURVE ( )  GEOMETRIC_REPRESENTATION_ITEM ( )  RATIONAL_B_SPLINE_CURVE ( ( 1.000000000000000000, 0.9238795325112867385, 1.000000000000000000, 0.9238795325112867385, 1.000000000000000000, 0.9238795325112867385, 1.000000000000000000, 0.9238795325112871826, 0.9999999999999995559 ) ) 
 REPRESENTATION_ITEM ( '' )  );
#12147=CARTESIAN_POINT ( 'NONE',  ( 2.066987300000001415, 64.00000000000000000, 49.15000000109247225 ) ) ;
#12156=CARTESIAN_POINT ( 'NONE',  ( 1.767766952966369987, 65.76776695296638309, 46.49999999999999289 ) ) ;
#12168=CARTESIAN_POINT ( 'NONE',  ( 32.50000000000000000, 52.00000000000000711, 15.00000000000000000 ) ) ;
#12174=DIRECTION ( 'NONE',  ( 1.000000000000000000, 0.000000000000000000, 0.000000000000000000 ) ) ;
#12177=CARTESIAN_POINT ( 'NONE',  ( 0.000000000000000000, 64.00000000000000000, 49.99999999999999289 ) ) ;
#12189=AXIS2_PLACEMENT_3D ( 'NONE', #6710, #444, #6429 ) ;
#12190=VECTOR ( 'NONE', #17045, 1000.000000000000000 ) ;
#12194=CARTESIAN_POINT ( 'NONE',  ( 2.500000000000001776, 65.03553390593273775, 47.35000000218494165 ) ) ;
#12201=VECTOR ( 'NONE', #19226, 1000.000000000000000 ) ;
#12204=CARTESIAN_POINT ( 'NONE',  ( 1.461580736456473906, 62.53841926354353120, 49.25000000109246656 ) ) ;
#12206=CARTESIAN_POINT ( 'NONE',  ( -4.000000000000001776, 67.00000000000000000, 34.99999999999999289 ) ) ;
#12208=CARTESIAN_POINT ( 'NONE',  ( 2.500000000000001776, 64.00000000000000000, 48.79999999999999716 ) ) ;
#12219=CARTESIAN_POINT ( 'NONE',  ( -1.265664690411616068E-16, 66.06698730000000808, 44.55000000109247082 ) ) ;
#12251=( BOUNDED_CURVE ( )  B_SPLINE_CURVE ( 2, ( #6873, #1178, #14512, #15892, #1082, #14613, #17554, #19127, #13129 ),
 .UNSPECIFIED., .F., .F. ) 
 B_SPLINE_CURVE_WITH_KNOTS ( ( 3, 2, 2, 2, 3 ),
 ( 0.1428571428571429047, 0.1607142857142857262, 0.1785714285714285476, 0.1964285714285713413, 0.2142857142857141350 ),
 .UNSPECIFIED. ) 
 CURVE ( )  GEOMETRIC_REPRESENTATION_ITEM ( )  RATIONAL_B_SPLINE_CURVE ( ( 0.9999999999999997780, 0.9238795325112869605, 1.000000000000000000, 0.9238795325112867385, 1.000000000000000000, 0.9238795325112867385, 1.000000000000000000, 0.9238795325112872936, 0.9999999999999994449 ) ) 
 REPRESENTATION_ITEM ( '' )  );
#12253=CARTESIAN_POINT ( 'NONE',  ( 0.8561741729129460632, 66.06698730000000808, 47.70000000109248361 ) ) ;
#12299=CARTESIAN_POINT ( 'NONE',  ( 4.592425496802577917E-16, 61.50000000000000000, 44.70000000218494307 ) ) ;
#12306=DIRECTION ( 'NONE',  ( -0.000000000000000000, -0.000000000000000000, -1.000000000000000000 ) ) ;
#12307=CARTESIAN_POINT ( 'NONE',  ( 3.796994071234847710E-16, 61.93301269999999903, 48.35000000109246798 ) ) ;
#12308=CARTESIAN_POINT ( 'NONE',  ( -15.00000000000000000, -0.000000000000000000, 37.00000000000000000 ) ) ;
#12310=EDGE_CURVE ( 'NONE', #297, #11681, #966, .T. ) ;
#12323=CARTESIAN_POINT ( 'NONE',  ( 2.066987300000002303, 63.14382582708705627, 46.70000000109248361 ) ) ;
#12329=ORIENTED_EDGE ( 'NONE', *, *, #11539, .T. ) ;
#12345=CARTESIAN_POINT ( 'NONE',  ( -1.461580736456473462, 62.53841926354353120, 48.85000000109246798 ) ) ;
#12346=DIRECTION ( 'NONE',  ( 0.000000000000000000, 0.000000000000000000, -1.000000000000000000 ) ) ;
#12355=FACE_BOUND ( 'NONE', #12664, .T. ) ;
#12385=CARTESIAN_POINT ( 'NONE',  ( 3.796994071234847710E-16, 61.93301269999999903, 45.15000000109247225 ) ) ;
#12393=CARTESIAN_POINT ( 'NONE',  ( 4.592425496802577917E-16, 61.50000000000000000, 47.10000000218494165 ) ) ;
#12404=CARTESIAN_POINT ( 'NONE',  ( 2.066987300000002303, 63.14382582708705627, 46.90000000109247225 ) ) ;
#12415=AXIS2_PLACEMENT_3D ( 'NONE', #12651, #14130, #13933 ) ;
#12417=ORIENTED_EDGE ( 'NONE', *, *, #6177, .F. ) ;
#12421=CARTESIAN_POINT ( 'NONE',  ( 0.8561741729129472844, 61.93301270000000613, 45.80000000109246372 ) ) ;
#12426=CARTESIAN_POINT ( 'NONE',  ( -14.99999999999999645, 52.00000000000000711, 20.99999999999998224 ) ) ;
#12443=CARTESIAN_POINT ( 'NONE',  ( -2.066987300000001415, 64.85617417291294373, 48.70000000109247651 ) ) ;
#12450=CYLINDRICAL_SURFACE ( 'NONE', #7568, 2.499999999999998668 ) ;
#12462=LINE ( 'NONE', #323, #2086 ) ;
#12463=ORIENTED_EDGE ( 'NONE', *, *, #2473, .T. ) ;
#12467=LINE ( 'NONE', #18470, #8736 ) ;
#12468=ORIENTED_EDGE ( 'NONE', *, *, #3737, .F. ) ;
#12474=CARTESIAN_POINT ( 'NONE',  ( -1.530808498934192803E-16, 66.50000000000000000, 45.90000000218494591 ) ) ;
#12485=CARTESIAN_POINT ( 'NONE',  ( 1.035533905932738197, 66.50000000000000000, 47.45000000218495018 ) ) ;
#12497=CARTESIAN_POINT ( 'NONE',  ( -0.8561741729129461742, 66.06698729999999387, 48.00000000109246656 ) ) ;
#12503=DIRECTION ( 'NONE',  ( -0.000000000000000000, -1.000000000000000000, -0.000000000000000000 ) ) ;
#12508=EDGE_CURVE ( 'NONE', #11681, #17737, #7160, .T. ) ;
#12510=EDGE_CURVE ( 'NONE', #3632, #9208, #4326, .T. ) ;
#12516=CARTESIAN_POINT ( 'NONE',  ( -0.8561741729129465073, 61.93301270000000613, 47.30000000109247082 ) ) ;
#12521=CARTESIAN_POINT ( 'NONE',  ( 24.00000000000000000, 0.000000000000000000, -67.72004514666936359 ) ) ;
#12523=AXIS2_PLACEMENT_3D ( 'NONE', #13719, #4, #11958 ) ;
#12525=LINE ( 'NONE', #11048, #12190 ) ;
#12544=EDGE_LOOP ( 'NONE', ( #16860, #15689 ) ) ;
#12590=CARTESIAN_POINT ( 'NONE',  ( 1.035533905932739751, 61.50000000000000000, 46.35000000218493454 ) ) ;
#12599=CARTESIAN_POINT ( 'NONE',  ( -1.265664690411616068E-16, 66.06698730000000808, 44.75000000109247367 ) ) ;
#12601=CARTESIAN_POINT ( 'NONE',  ( -2.500000000000003109, 65.03553390593272354, 48.45000000218494307 ) ) ;
#12608=CARTESIAN_POINT ( 'NONE',  ( 0.8561741729129471734, 61.93301270000000613, 45.00000000109247367 ) ) ;
#12612=CARTESIAN_POINT ( 'NONE',  ( 2.066987300000001859, 64.85617417291294373, 47.60000000109246798 ) ) ;
#12618=CARTESIAN_POINT ( 'NONE',  ( -2.500000000000001776, 64.00000000000000000, 49.99999999999999289 ) ) ;
#12629=ORIENTED_EDGE ( 'NONE', *, *, #8564, .F. ) ;
#12638=DIRECTION ( 'NONE',  ( -0.000000000000000000, 1.000000000000000000, -0.000000000000000000 ) ) ;
#12651=CARTESIAN_POINT ( 'NONE',  ( 32.50000000000000000, 52.00000000000000711, -35.00000000000000000 ) ) ;
#12659=DIRECTION ( 'NONE',  ( -0.000000000000000000, -0.000000000000000000, -1.000000000000000000 ) ) ;
#12664=EDGE_LOOP ( 'NONE', ( #16097, #18290 ) ) ;
#12669=CARTESIAN_POINT ( 'NONE',  ( -2.500000000000011546, 65.03553390593272354, 46.05000000218494449 ) ) ;
#12678=CARTESIAN_POINT ( 'NONE',  ( -2.066987300000001415, 63.14382582708705627, 47.20000000109248361 ) ) ;
#12686=CARTESIAN_POINT ( 'NONE',  ( -2.500000000000001776, 64.00000000000000000, 49.19999999999999574 ) ) ;
#12689=VECTOR ( 'NONE', #14352, 1000.000000000000000 ) ;
#12701=CARTESIAN_POINT ( 'NONE',  ( 2.066987300000001859, 64.85617417291294373, 46.80000000109246372 ) ) ;
#12703=CARTESIAN_POINT ( 'NONE',  ( -4.000000000000001776, 67.00000000000000000, 30.00000000000000000 ) ) ;
#12710=CARTESIAN_POINT ( 'NONE',  ( 1.035533905932739751, 61.50000000000000000, 48.64999999999999858 ) ) ;
#12722=EDGE_CURVE ( 'NONE', #964, #7747, #211, .T. ) ;
#12723=CARTESIAN_POINT ( 'NONE',  ( 2.500000000000006661, 65.03553390593272354, 47.24999999999998579 ) ) ;
#12732=CARTESIAN_POINT ( 'NONE',  ( -10.00000000000000000, 35.00000000000000000, 0.000000000000000000 ) ) ;
#12740=DIRECTION ( 'NONE',  ( 1.000000000000000000, 0.000000000000000000, 0.000000000000000000 ) ) ;
#12755=ORIENTED_EDGE ( 'NONE', *, *, #8564, .T. ) ;
#12767=CARTESIAN_POINT ( 'NONE',  ( -2.066987300000001415, 63.14382582708705627, 46.40000000109246514 ) ) ;
#12777=CARTESIAN_POINT ( 'NONE',  ( -1.767766952966369765, 62.23223304703363112, 49.29999999999999716 ) ) ;
#12785=CARTESIAN_POINT ( 'NONE',  ( 0.8561741729129460632, 66.06698730000000808, 45.30000000109246372 ) ) ;
#12790=CARTESIAN_POINT ( 'NONE',  ( -2.066987300000001415, 63.14382582708705627, 48.20000000109247651 ) ) ;
#12806=AXIS2_PLACEMENT_3D ( 'NONE', #14190, #6737, #17232 ) ;
#12825=EDGE_CURVE ( 'NONE', #14815, #2308, #17528, .T. ) ;
#12826=VECTOR ( 'NONE', #16278, 1000.000000000000000 ) ;
#12843=( LENGTH_UNIT ( ) NAMED_UNIT ( * ) SI_UNIT ( .MILLI., .METRE. ) );
#12858=CYLINDRICAL_SURFACE ( 'NONE', #9885, 2.500000000000002220 ) ;
#12865=CARTESIAN_POINT ( 'NONE',  ( 2.066987300000002303, 63.14382582708705627, 48.30000000109247082 ) ) ;
#12867=( BOUNDED_CURVE ( )  B_SPLINE_CURVE ( 2, ( #720, #12669, #3468, #9444, #12474, #2284, #6700, #18670, #8269 ),
 .UNSPECIFIED., .F., .F. ) 
 B_SPLINE_CURVE_WITH_KNOTS ( ( 3, 2, 2, 2, 3 ),
 ( 0.5714285714285711748, 0.5892857142857141906, 0.6071428571428569843, 0.6250000000000000000, 0.6428571428571429047 ),
 .UNSPECIFIED. ) 
 CURVE ( )  GEOMETRIC_REPRESENTATION_ITEM ( )  RATIONAL_B_SPLINE_CURVE ( ( 1.000000000000000888, 0.9238795325112857393, 1.000000000000000000, 0.9238795325112867385, 1.000000000000000000, 0.9238795325112867385, 1.000000000000000000, 0.9238795325112867385, 1.000000000000000000 ) ) 
 REPRESENTATION_ITEM ( '' )  );
#12878=CARTESIAN_POINT ( 'NONE',  ( -1.461580736456473906, 65.46158073645646880, 45.65000000109247225 ) ) ;
#12886=DIRECTION ( 'NONE',  ( 1.000000000000000000, 0.000000000000000000, 0.000000000000000000 ) ) ;
#12890=CARTESIAN_POINT ( 'NONE',  ( -2.066987300000001415, 64.00000000000000000, 48.95000000109246940 ) ) ;
#12898=VECTOR ( 'NONE', #4503, 1000.000000000000000 ) ;
#12904=( LENGTH_UNIT ( ) NAMED_UNIT ( * ) SI_UNIT ( .MILLI., .METRE. ) );
#12919=FACE_OUTER_BOUND ( 'NONE', #14378, .T. ) ;
#12933=CARTESIAN_POINT ( 'NONE',  ( -1.530808498934192803E-16, 66.50000000000000000, 45.79999999999999005 ) ) ;
#12938=CARTESIAN_POINT ( 'NONE',  ( 1.035533905932738197, 66.50000000000000000, 46.65000000218494591 ) ) ;
#12939=ORIENTED_EDGE ( 'NONE', *, *, #12508, .T. ) ;
#12953=CARTESIAN_POINT ( 'NONE',  ( -1.265664690411616068E-16, 66.06698730000000808, 47.75000000109246656 ) ) ;
#12957=EDGE_LOOP ( 'NONE', ( #16949, #459 ) ) ;
#12967=CARTESIAN_POINT ( 'NONE',  ( -2.066987300000001415, 64.00000000000000000, 44.95000000109246940 ) ) ;
#12968=CARTESIAN_POINT ( 'NONE',  ( -2.066987300000000971, 63.14382582708704916, 49.00000000109246656 ) ) ;
#12969=CARTESIAN_POINT ( 'NONE',  ( -1.767766952966369765, 62.23223304703363112, 48.60000000218494165 ) ) ;
#12975=CARTESIAN_POINT ( 'NONE',  ( 3.796994071234847710E-16, 61.93301269999999903, 45.75000000109247367 ) ) ;
#12977=DIRECTION ( 'NONE',  ( 0.000000000000000000, 1.000000000000000000, 0.000000000000000000 ) ) ;
#12980=CARTESIAN_POINT ( 'NONE',  ( -2.066987300000001859, 64.85617417291294373, 44.70000000109248361 ) ) ;
#12982=CARTESIAN_POINT ( 'NONE',  ( -15.00000000000000000, 0.000000000000000000, 33.99999999999999289 ) ) ;
#12987=CYLINDRICAL_SURFACE ( 'NONE', #19123, 2.499999999999998668 ) ;
#12994=VECTOR ( 'NONE', #14496, 1000.000000000000000 ) ;
#13004=ORIENTED_EDGE ( 'NONE', *, *, #12310, .T. ) ;
#13006=VERTEX_POINT ( 'NONE', #16724 ) ;
#13015=CIRCLE ( 'NONE', #10185, 2.999999999999999112 ) ;
#13023=DIRECTION ( 'NONE',  ( -1.000000000000000000, 0.000000000000000000, 0.000000000000000000 ) ) ;
#13027=CIRCLE ( 'NONE', #7403, 2.500000000000001776 ) ;
#13028=CARTESIAN_POINT ( 'NONE',  ( -1.035533905932738641, 66.50000000000000000, 45.04999999999999005 ) ) ;
#13032=CARTESIAN_POINT ( 'NONE',  ( 2.499999999999999112, 65.03553390593273775, 46.55000000218494449 ) ) ;
#13033=ORIENTED_EDGE ( 'NONE', *, *, #3850, .T. ) ;
#13038=( GEOMETRIC_REPRESENTATION_CONTEXT ( 3 ) GLOBAL_UNCERTAINTY_ASSIGNED_CONTEXT ( ( #8274 ) ) GLOBAL_UNIT_ASSIGNED_CONTEXT ( ( #12904, #17144, #3993 ) ) REPRESENTATION_CONTEXT ( 'NONE', 'WORKASPACE' ) );
#13046=CARTESIAN_POINT ( 'NONE',  ( -2.066987300000001415, 64.00000000000000000, 47.15000000109247225 ) ) ;
#13052=CARTESIAN_POINT ( 'NONE',  ( -2.500000000000001776, 64.00000000000000000, 46.10000000218494165 ) ) ;
#13056=CARTESIAN_POINT ( 'NONE',  ( 4.000000000000000888, 52.00000000000000711, 30.00000000000000000 ) ) ;
#13060=CARTESIAN_POINT ( 'NONE',  ( 2.500000000000001776, 65.03553390593273775, 48.04999999999999716 ) ) ;
#13061=CARTESIAN_POINT ( 'NONE',  ( -1.461580736456473462, 62.53841926354353120, 49.05000000109247082 ) ) ;
#13072=CARTESIAN_POINT ( 'NONE',  ( 3.796994071234847710E-16, 61.93301269999999903, 47.55000000109247082 ) ) ;
#13077=CARTESIAN_POINT ( 'NONE',  ( -2.066987300000001415, 64.00000000000000000, 49.75000000109246656 ) ) ;
#13097=CIRCLE ( 'NONE', #13745, 2.999999999999999112 ) ;
#13101=EDGE_LOOP ( 'NONE', ( #18714, #11430, #2783, #1149 ) ) ;
#13102=CARTESIAN_POINT ( 'NONE',  ( -1.035533905932738863, 61.50000000000000000, 46.95000000000000284 ) ) ;
#13113=CARTESIAN_POINT ( 'NONE',  ( 1.035533905932739751, 61.50000000000000000, 47.15000000218494591 ) ) ;
#13121=ORIENTED_EDGE ( 'NONE', *, *, #1876, .T. ) ;
#13129=CARTESIAN_POINT ( 'NONE',  ( 2.500000000000001776, 64.00000000000000000, 48.79999999999999716 ) ) ;
#13151=CARTESIAN_POINT ( 'NONE',  ( -0.8561741729129461742, 66.06698729999999387, 46.20000000109247651 ) ) ;
#13160=AXIS2_PLACEMENT_3D ( 'NONE', #8878, #16638, #8778 ) ;
#13163=CARTESIAN_POINT ( 'NONE',  ( 2.500000000000001776, 65.03553390593273775, 46.45000000000000284 ) ) ;
#13164=CARTESIAN_POINT ( 'NONE',  ( -2.066987300000001415, 64.00000000000000000, 49.75000000109246656 ) ) ;
#13170=CIRCLE ( 'NONE', #3169, 2.499999999999998668 ) ;
#13175=FACE_OUTER_BOUND ( 'NONE', #2253, .T. ) ;
#13179=CARTESIAN_POINT ( 'NONE',  ( 2.066987300000001415, 64.00000000000000000, 46.95000000109246940 ) ) ;
#13184=FACE_OUTER_BOUND ( 'NONE', #9325, .T. ) ;
#13196=VERTEX_POINT ( 'NONE', #4964 ) ;
#13205=CARTESIAN_POINT ( 'NONE',  ( -2.500000000000001776, 64.00000000000000000, 46.79999999999999716 ) ) ;
#13206=ORIENTED_EDGE ( 'NONE', *, *, #1942, .T. ) ;
#13211=PLANE ( 'NONE',  #19070 ) ;
#13215=CARTESIAN_POINT ( 'NONE',  ( -32.50000000000000000, 52.00000000000000711, -32.50000000000000000 ) ) ;
#13216=CARTESIAN_POINT ( 'NONE',  ( 1.767766952966370653, 62.23223304703363112, 47.20000000218494307 ) ) ;
#13223=VERTEX_POINT ( 'NONE', #18493 ) ;
#13226=CARTESIAN_POINT ( 'NONE',  ( -4.000000000000001776, 67.00000000000000000, 34.99999999999999289 ) ) ;
#13230=VERTEX_POINT ( 'NONE', #18586 ) ;
#13238=CARTESIAN_POINT ( 'NONE',  ( -15.00000000000000000, 35.00000000000000000, 33.99999999999999289 ) ) ;
#13247=CARTESIAN_POINT ( 'NONE',  ( -1.461580736456473462, 62.53841926354353120, 44.85000000109246798 ) ) ;
#13255=CARTESIAN_POINT ( 'NONE',  ( 1.767766952966370653, 62.23223304703363112, 45.50000000000000000 ) ) ;
#13259=CARTESIAN_POINT ( 'NONE',  ( -1.035533905932738863, 61.50000000000000000, 47.74999999999999289 ) ) ;
#13260=CARTESIAN_POINT ( 'NONE',  ( -1.461580736456473906, 65.46158073645646880, 47.25000000109246656 ) ) ;
#13265=EDGE_CURVE ( 'NONE', #19297, #9711, #5153, .T. ) ;
#13269=CARTESIAN_POINT ( 'NONE',  ( -0.8561741729129465073, 61.93301270000000613, 45.10000000109246798 ) ) ;
#13273=DIRECTION ( 'NONE',  ( -0.000000000000000000, -1.000000000000000000, -0.000000000000000000 ) ) ;
#13296=VERTEX_POINT ( 'NONE', #1923 ) ;
#13298=ADVANCED_FACE ( 'NONE', ( #11114 ), #13967, .T. ) ;
#13320=DIRECTION ( 'NONE',  ( -0.000000000000000000, -0.000000000000000000, -1.000000000000000000 ) ) ;
#13324=AXIS2_PLACEMENT_3D ( 'NONE', #14473, #11421, #9676 ) ;
#13325=CARTESIAN_POINT ( 'NONE',  ( -1.530808498934192803E-16, 66.50000000000000000, 47.50000000218494023 ) ) ;
#13326=ORIENTED_EDGE ( 'NONE', *, *, #2336, .F. ) ;
#13337=CARTESIAN_POINT ( 'NONE',  ( -1.530808498934192803E-16, 66.50000000000000000, 48.19999999999999574 ) ) ;
#13341=DIRECTION ( 'NONE',  ( 0.000000000000000000, 0.000000000000000000, 1.000000000000000000 ) ) ;
#13346=PRODUCT_DEFINITION_CONTEXT ( 'detailed design', #14448, 'design' ) ;
#13349=CARTESIAN_POINT ( 'NONE',  ( 0.8561741729129472844, 61.93301270000000613, 45.00000000109246656 ) ) ;
#13359=CARTESIAN_POINT ( 'NONE',  ( 2.500000000000001776, 64.00000000000000000, 44.90000000218493881 ) ) ;
#13362=CARTESIAN_POINT ( 'NONE',  ( 0.8561741729129471734, 61.93301270000000613, 46.80000000109247082 ) ) ;
#13373=CARTESIAN_POINT ( 'NONE',  ( 1.461580736456473906, 62.53841926354353120, 46.05000000109246372 ) ) ;
#13380=CARTESIAN_POINT ( 'NONE',  ( 24.00000000000000000, 47.00000000000000711, 18.00000000000000000 ) ) ;
#13382=DIRECTION ( 'NONE',  ( 0.000000000000000000, -1.000000000000000000, 0.000000000000000000 ) ) ;
#13393=CARTESIAN_POINT ( 'NONE',  ( 1.461580736456473684, 65.46158073645646880, 48.45000000109247651 ) ) ;
#13396=ORIENTED_EDGE ( 'NONE', *, *, #5566, .T. ) ;
#13398=CARTESIAN_POINT ( 'NONE',  ( -2.500000000000001776, 62.96446609406726225, 46.84999999999998721 ) ) ;
#13401=DIRECTION ( 'NONE',  ( 0.000000000000000000, 0.000000000000000000, 1.000000000000000000 ) ) ;
#13408=ORIENTED_EDGE ( 'NONE', *, *, #16636, .T. ) ;
#13443=CIRCLE ( 'NONE', #3446, 2.999999999999999112 ) ;
#13444=CARTESIAN_POINT ( 'NONE',  ( 1.461580736456473684, 65.46158073645646880, 45.25000000109247367 ) ) ;
#13447=ORIENTED_EDGE ( 'NONE', *, *, #19188, .F. ) ;
#13451=CARTESIAN_POINT ( 'NONE',  ( 14.99999999999998579, 73.00000000000001421, 20.99999999999997513 ) ) ;
#13452=CARTESIAN_POINT ( 'NONE',  ( -32.50000000000000000, 52.00000000000000711, -32.50000000000000000 ) ) ;
#13457=VECTOR ( 'NONE', #17477, 1000.000000000000000 ) ;
#13458=CARTESIAN_POINT ( 'NONE',  ( 0.8561741729129471734, 61.93301270000000613, 48.40000000109247225 ) ) ;
#13468=VECTOR ( 'NONE', #11563, 1000.000000000000000 ) ;
#13474=CARTESIAN_POINT ( 'NONE',  ( -1.461580736456473906, 65.46158073645646880, 44.85000000109246798 ) ) ;
#13488=VECTOR ( 'NONE', #6050, 1000.000000000000000 ) ;
#13490=EDGE_LOOP ( 'NONE', ( #9528, #10167 ) ) ;
#13493=FACE_OUTER_BOUND ( 'NONE', #1181, .T. ) ;
#13501=CARTESIAN_POINT ( 'NONE',  ( -1.530808498934192803E-16, 66.50000000000000000, 45.00000000000000000 ) ) ;
#13513=DIRECTION ( 'NONE',  ( 0.000000000000000000, 0.000000000000000000, 1.000000000000000000 ) ) ;
#13515=CARTESIAN_POINT ( 'NONE',  ( 3.999999999999998224, 67.00000000000000000, 30.00000000000000000 ) ) ;
#13516=VERTEX_POINT ( 'NONE', #16507 ) ;
#13526=CARTESIAN_POINT ( 'NONE',  ( -2.500000000000001776, 64.00000000000000000, 45.19999999999999574 ) ) ;
#13529=ORIENTED_EDGE ( 'NONE', *, *, #15515, .F. ) ;
#13540=CARTESIAN_POINT ( 'NONE',  ( 1.767766952966369987, 65.76776695296638309, 48.09999999999999432 ) ) ;
#13549=VERTEX_POINT ( 'NONE', #13452 ) ;
#13555=CARTESIAN_POINT ( 'NONE',  ( 0.000000000000000000, 52.00000000000000711, -67.72004514666936359 ) ) ;
#13557=CARTESIAN_POINT ( 'NONE',  ( -2.066987300000001415, 64.00000000000000000, 46.55000000109247082 ) ) ;
#13566=CARTESIAN_POINT ( 'NONE',  ( 1.035533905932738197, 66.50000000000000000, 49.05000000218495160 ) ) ;
#13575=CARTESIAN_POINT ( 'NONE',  ( -0.8561741729129465073, 61.93301270000000613, 46.70000000109248361 ) ) ;
#13579=FACE_OUTER_BOUND ( 'NONE', #14317, .T. ) ;
#13583=EDGE_LOOP ( 'NONE', ( #195, #6284, #8907, #2839, #11559, #3420 ) ) ;
#13587=DIRECTION ( 'NONE',  ( 0.000000000000000000, -0.000000000000000000, -1.000000000000000000 ) ) ;
#13591=CARTESIAN_POINT ( 'NONE',  ( -41.00000000000000000, 52.00000000000000711, -67.72004514666936359 ) ) ;
#13617=( BOUNDED_CURVE ( )  B_SPLINE_CURVE ( 2, ( #17953, #1285, #18054, #10483, #13325, #108, #7262, #4324, #12055 ),
 .UNSPECIFIED., .F., .F. ) 
 B_SPLINE_CURVE_WITH_KNOTS ( ( 3, 2, 2, 2, 3 ),
 ( 0.2857142857142859205, 0.3035714285714287142, 0.3214285714285715634, 0.3392857142857143571, 0.3571428571428571508 ),
 .UNSPECIFIED. ) 
 CURVE ( )  GEOMETRIC_REPRESENTATION_ITEM ( )  RATIONAL_B_SPLINE_CURVE ( ( 0.9999999999999990008, 0.9238795325112877377, 1.000000000000000000, 0.9238795325112867385, 1.000000000000000000, 0.9238795325112867385, 1.000000000000000000, 0.9238795325112867385, 1.000000000000000000 ) ) 
 REPRESENTATION_ITEM ( '' )  );
#13618=CARTESIAN_POINT ( 'NONE',  ( -2.066987300000001415, 64.85617417291294373, 47.90000000109247225 ) ) ;
#13619=DIRECTION ( 'NONE',  ( -0.000000000000000000, 1.000000000000000000, -0.000000000000000000 ) ) ;
#13636=CARTESIAN_POINT ( 'NONE',  ( 0.000000000000000000, 64.00000000000000000, 49.99999999999999289 ) ) ;
#13663=CARTESIAN_POINT ( 'NONE',  ( 1.767766952966369987, 65.76776695296638309, 48.20000000218494307 ) ) ;
#13667=CARTESIAN_POINT ( 'NONE',  ( -2.066987300000001415, 64.00000000000000000, 46.55000000109247082 ) ) ;
#13673=LINE ( 'NONE', #11731, #5708 ) ;
#13674=CARTESIAN_POINT ( 'NONE',  ( 1.461580736456473684, 65.46158073645646880, 46.25000000109246656 ) ) ;
#13691=PLANE ( 'NONE',  #5812 ) ;
#13705=DIRECTION ( 'NONE',  ( -0.000000000000000000, -1.000000000000000000, -0.000000000000000000 ) ) ;
#13711=EDGE_CURVE ( 'NONE', #17737, #18430, #19006, .T. ) ;
#13713=CARTESIAN_POINT ( 'NONE',  ( 0.000000000000000000, 0.000000000000000000, 0.000000000000000000 ) ) ;
#13718=CARTESIAN_POINT ( 'NONE',  ( 1.461580736456473906, 62.53841926354353120, 49.05000000109247082 ) ) ;
#13719=CARTESIAN_POINT ( 'NONE',  ( -32.50000000000000000, 47.00000000000000711, -35.00000000000000000 ) ) ;
#13730=CARTESIAN_POINT ( 'NONE',  ( -41.00000000000000000, 47.00000000000000711, 18.00000000000000000 ) ) ;
#13745=AXIS2_PLACEMENT_3D ( 'NONE', #16924, #9356, #7802 ) ;
#13755=CIRCLE ( 'NONE', #917, 2.500000000000001776 ) ;
#13760=VECTOR ( 'NONE', #6071, 1000.000000000000000 ) ;
#13762=ORIENTED_EDGE ( 'NONE', *, *, #11381, .F. ) ;
#13765=AXIS2_PLACEMENT_3D ( 'NONE', #6192, #17750, #9016 ) ;
#13766=CARTESIAN_POINT ( 'NONE',  ( 2.500000000000001776, 65.03553390593273775, 44.95000000218494307 ) ) ;
#13776=CARTESIAN_POINT ( 'NONE',  ( 2.066987300000001415, 64.00000000000000000, 48.55000000109247082 ) ) ;
#13780=DIRECTION ( 'NONE',  ( -0.000000000000000000, -0.000000000000000000, -1.000000000000000000 ) ) ;
#13800=ORIENTED_EDGE ( 'NONE', *, *, #11039, .F. ) ;
#13819=EDGE_CURVE ( 'NONE', #17611, #4643, #18473, .T. ) ;
#13821=CARTESIAN_POINT ( 'NONE',  ( -1.461580736456473906, 65.46158073645646880, 48.65000000109247225 ) ) ;
#13822=DIRECTION ( 'NONE',  ( 0.000000000000000000, 0.000000000000000000, -1.000000000000000000 ) ) ;
#13833=PLANE ( 'NONE',  #15817 ) ;
#13837=CARTESIAN_POINT ( 'NONE',  ( -1.530808498934192803E-16, 66.50000000000000000, 49.10000000218494165 ) ) ;
#13840=CARTESIAN_POINT ( 'NONE',  ( 0.000000000000000000, 64.00000000000000000, 49.99999999999999289 ) ) ;
#13852=LINE ( 'NONE', #7980, #6255 ) ;
#13855=CARTESIAN_POINT ( 'NONE',  ( 2.500000000000007105, 62.96446609406726225, 46.34999999999998721 ) ) ;
#13866=CARTESIAN_POINT ( 'NONE',  ( -1.035533905932738863, 61.50000000000000000, 47.05000000218494449 ) ) ;
#13875=CARTESIAN_POINT ( 'NONE',  ( 2.066987300000001859, 64.85617417291294373, 47.00000000109246656 ) ) ;
#13881=ADVANCED_FACE ( 'NONE', ( #18280 ), #10806, .T. ) ;
#13888=LINE ( 'NONE', #11356, #12994 ) ;
#13890=CARTESIAN_POINT ( 'NONE',  ( 0.8561741729129460632, 66.06698729999999387, 46.10000000109246798 ) ) ;
#13897=LINE ( 'NONE', #12618, #9682 ) ;
#13913=CARTESIAN_POINT ( 'NONE',  ( 2.066987300000001859, 63.14382582708704916, 49.10000000109246088 ) ) ;
#13919=ORIENTED_EDGE ( 'NONE', *, *, #1576, .T. ) ;
#13924=FACE_OUTER_BOUND ( 'NONE', #2622, .T. ) ;
#13933=DIRECTION ( 'NONE',  ( 0.000000000000000000, 0.000000000000000000, 1.000000000000000000 ) ) ;
#13952=DIRECTION ( 'NONE',  ( -1.000000000000000000, 0.000000000000000000, 0.000000000000000000 ) ) ;
#13963=CARTESIAN_POINT ( 'NONE',  ( -1.035533905932738641, 66.50000000000000000, 45.15000000218493881 ) ) ;
#13967=CYLINDRICAL_SURFACE ( 'NONE', #15808, 2.500000000000001776 ) ;
#13970=DIRECTION ( 'NONE',  ( -0.000000000000000000, 1.000000000000000000, -0.000000000000000000 ) ) ;
#13974=CARTESIAN_POINT ( 'NONE',  ( 2.066987300000001859, 64.85617417291294373, 48.60000000109246798 ) ) ;
#13977=CARTESIAN_POINT ( 'NONE',  ( 2.500000000000001776, 64.00000000000000000, 49.99999999999999289 ) ) ;
#13984=AXIS2_PLACEMENT_3D ( 'NONE', #15217, #9132, #10691 ) ;
#13990=CARTESIAN_POINT ( 'NONE',  ( -1.265664690411616068E-16, 66.06698730000000808, 46.95000000109246940 ) ) ;
#13991=FACE_OUTER_BOUND ( 'NONE', #18435, .T. ) ;
#13992=VERTEX_POINT ( 'NONE', #3848 ) ;
#13997=CARTESIAN_POINT ( 'NONE',  ( 24.00000000000000000, -0.000000000000000000, 18.00000000000000000 ) ) ;
#14001=ORIENTED_EDGE ( 'NONE', *, *, #13819, .F. ) ;
#14006=ORIENTED_EDGE ( 'NONE', *, *, #16089, .T. ) ;
#14012=CYLINDRICAL_SURFACE ( 'NONE', #318, 2.999999999999999112 ) ;
#14028=( BOUNDED_CURVE ( )  B_SPLINE_CURVE ( 2, ( #7463, #6007, #17963, #18650, #6495, #1887, #17078, #15698, #5025 ),
 .UNSPECIFIED., .F., .F. ) 
 B_SPLINE_CURVE_WITH_KNOTS ( ( 3, 2, 2, 2, 3 ),
 ( 0.000000000000000000, 0.01785714285714280411, 0.03571428571428560822, 0.05357142857142841580, 0.07142857142857121644 ),
 .UNSPECIFIED. ) 
 CURVE ( )  GEOMETRIC_REPRESENTATION_ITEM ( )  RATIONAL_B_SPLINE_CURVE ( ( 1.000000000000000000, 0.9238795325112867385, 1.000000000000000000, 0.9238795325112867385, 1.000000000000000000, 0.9238795325112867385, 1.000000000000000000, 0.9238795325112876267, 0.9999999999999991118 ) ) 
 REPRESENTATION_ITEM ( '' )  );
#14029=CARTESIAN_POINT ( 'NONE',  ( 2.500000000000001776, 64.00000000000000000, 48.10000000218494165 ) ) ;
#14031=VERTEX_POINT ( 'NONE', #9905 ) ;
#14039=DIRECTION ( 'NONE',  ( 0.000000000000000000, 0.000000000000000000, -1.000000000000000000 ) ) ;
#14047=CARTESIAN_POINT ( 'NONE',  ( -1.461580736456473462, 62.53841926354353120, 45.05000000109246372 ) ) ;
#14048=EDGE_CURVE ( 'NONE', #3539, #375, #1090, .T. ) ;
#14057=CARTESIAN_POINT ( 'NONE',  ( 1.767766952966370653, 62.23223304703363112, 47.20000000218494307 ) ) ;
#14069=CARTESIAN_POINT ( 'NONE',  ( 3.796994071234847710E-16, 61.93301269999999903, 45.95000000109246940 ) ) ;
#14077=ORIENTED_EDGE ( 'NONE', *, *, #18128, .T. ) ;
#14088=CARTESIAN_POINT ( 'NONE',  ( 3.796994071234847710E-16, 61.93301269999999903, 47.35000000109246798 ) ) ;
#14089=EDGE_LOOP ( 'NONE', ( #7643, #18012, #18122 ) ) ;
#14095=FACE_OUTER_BOUND ( 'NONE', #9495, .T. ) ;
#14112=CARTESIAN_POINT ( 'NONE',  ( 1.767766952966369987, 65.76776695296638309, 47.29999999999999716 ) ) ;
#14122=FACE_OUTER_BOUND ( 'NONE', #3750, .T. ) ;
#14123=CARTESIAN_POINT ( 'NONE',  ( -1.767766952966369765, 62.23223304703363112, 45.29999999999999005 ) ) ;
#14130=DIRECTION ( 'NONE',  ( -0.000000000000000000, -1.000000000000000000, -0.000000000000000000 ) ) ;
#14134=CIRCLE ( 'NONE', #13160, 2.500000000000002220 ) ;
#14143=DIRECTION ( 'NONE',  ( -1.000000000000000000, -0.000000000000000000, -0.000000000000000000 ) ) ;
#14147=( BOUNDED_CURVE ( )  B_SPLINE_CURVE ( 2, ( #3815, #15583, #2151, #8139, #6211, #771, #14112, #12723, #17335 ),
 .UNSPECIFIED., .F., .F. ) 
 B_SPLINE_CURVE_WITH_KNOTS ( ( 3, 2, 2, 2, 3 ),
 ( 0.4285714285714284921, 0.4464285714285714524, 0.4642857142857143016, 0.4821428571428572063, 0.5000000000000001110 ),
 .UNSPECIFIED. ) 
 CURVE ( )  GEOMETRIC_REPRESENTATION_ITEM ( )  RATIONAL_B_SPLINE_CURVE ( ( 1.000000000000000222, 0.9238795325112865164, 1.000000000000000000, 0.9238795325112867385, 1.000000000000000000, 0.9238795325112867385, 1.000000000000000000, 0.9238795325112862944, 1.000000000000000444 ) ) 
 REPRESENTATION_ITEM ( '' )  );
#14156=VECTOR ( 'NONE', #5109, 1000.000000000000000 ) ;
#14158=CARTESIAN_POINT ( 'NONE',  ( -1.767766952966369765, 62.23223304703363112, 47.00000000218494733 ) ) ;
#14162=CARTESIAN_POINT ( 'NONE',  ( 0.000000000000000000, 52.00000000000000711, 30.00000000000000000 ) ) ;
#14168=CARTESIAN_POINT ( 'NONE',  ( -1.767766952966369765, 62.23223304703363112, 48.49999999999999289 ) ) ;
#14180=DIRECTION ( 'NONE',  ( 0.000000000000000000, 0.000000000000000000, 1.000000000000000000 ) ) ;
#14184=CARTESIAN_POINT ( 'NONE',  ( 1.461580736456473906, 62.53841926354353120, 46.65000000109247225 ) ) ;
#14188=CARTESIAN_POINT ( 'NONE',  ( -2.500000000000001776, 64.00000000000000000, 46.90000000218494591 ) ) ;
#14190=CARTESIAN_POINT ( 'NONE',  ( 0.000000000000000000, 64.00000000000000000, 49.99999999999999289 ) ) ;
#14215=CARTESIAN_POINT ( 'NONE',  ( 0.000000000000000000, 64.00000000000000000, 49.99999999999999289 ) ) ;
#14228=AXIS2_PLACEMENT_3D ( 'NONE', #17891, #11893, #17684 ) ;
#14243=DIRECTION ( 'NONE',  ( 2.602085213965211135E-16, -1.000000000000000000, 0.000000000000000000 ) ) ;
#14247=CARTESIAN_POINT ( 'NONE',  ( 0.8561741729129460632, 66.06698729999999387, 47.70000000109248361 ) ) ;
#14256=CARTESIAN_POINT ( 'NONE',  ( -2.500000000000001776, 65.03553390593273775, 48.35000000000000142 ) ) ;
#14259=AXIS2_PLACEMENT_3D ( 'NONE', #10647, #16650, #8795 ) ;
#14267=CARTESIAN_POINT ( 'NONE',  ( -0.8561741729129466183, 61.93301270000000613, 44.90000000109247225 ) ) ;
#14269=PLANE ( 'NONE',  #8221 ) ;
#14274=CARTESIAN_POINT ( 'NONE',  ( 2.066987300000001859, 64.85617417291294373, 45.20000000109248361 ) ) ;
#14281=CARTESIAN_POINT ( 'NONE',  ( 2.500000000000007994, 62.96446609406726225, 48.74999999999999289 ) ) ;
#14294=FACE_OUTER_BOUND ( 'NONE', #16846, .T. ) ;
#14305=DIRECTION ( 'NONE',  ( -0.000000000000000000, -0.000000000000000000, -1.000000000000000000 ) ) ;
#14313=ORIENTED_EDGE ( 'NONE', *, *, #14048, .F. ) ;
#14317=EDGE_LOOP ( 'NONE', ( #11819, #19191, #7362, #11172 ) ) ;
#14322=ORIENTED_EDGE ( 'NONE', *, *, #9946, .F. ) ;
#14329=DIRECTION ( 'NONE',  ( 0.000000000000000000, 1.000000000000000000, -0.000000000000000000 ) ) ;
#14338=CARTESIAN_POINT ( 'NONE',  ( 2.066987300000001415, 64.00000000000000000, 49.15000000109247225 ) ) ;
#14348=CARTESIAN_POINT ( 'NONE',  ( 1.035533905932738197, 66.50000000000000000, 48.94999999999999574 ) ) ;
#14349=CARTESIAN_POINT ( 'NONE',  ( -2.066987300000001415, 64.85617417291294373, 48.90000000109247225 ) ) ;
#14352=DIRECTION ( 'NONE',  ( 0.000000000000000000, 1.000000000000000000, 0.000000000000000000 ) ) ;
#14357=ADVANCED_FACE ( 'NONE', ( #15304 ), #13833, .T. ) ;
#14359=FACE_OUTER_BOUND ( 'NONE', #5877, .T. ) ;
#14362=CARTESIAN_POINT ( 'NONE',  ( 2.066987300000002303, 63.14382582708705627, 49.30000000109246372 ) ) ;
#14370=CARTESIAN_POINT ( 'NONE',  ( -41.00000000000000000, 0.000000000000000000, 30.00000000000000000 ) ) ;
#14374=VERTEX_POINT ( 'NONE', #7627 ) ;
#14378=EDGE_LOOP ( 'NONE', ( #19327, #3551, #17723, #324 ) ) ;
#14394=EDGE_LOOP ( 'NONE', ( #8817, #10144, #3305, #11696 ) ) ;
#14409=ORIENTED_EDGE ( 'NONE', *, *, #15657, .T. ) ;
#14410=ADVANCED_FACE ( 'NONE', ( #80 ), #13691, .F. ) ;
#14412=EDGE_CURVE ( 'NONE', #2559, #908, #4689, .T. ) ;
#14419=VECTOR ( 'NONE', #8512, 1000.000000000000000 ) ;
#14438=CARTESIAN_POINT ( 'NONE',  ( -2.066987300000001415, 63.14382582708705627, 48.00000000109246656 ) ) ;
#14448=APPLICATION_CONTEXT ( 'automotive_design' ) ;
#14449=CARTESIAN_POINT ( 'NONE',  ( 2.500000000000002220, 62.96446609406726935, 48.74999999999999289 ) ) ;
#14452=EDGE_CURVE ( 'NONE', #15669, #4696, #10970, .T. ) ;
#14455=CARTESIAN_POINT ( 'NONE',  ( -14.99999999999999645, 73.00000000000001421, 26.99999999999997868 ) ) ;
#14459=CARTESIAN_POINT ( 'NONE',  ( 2.066987300000001859, 63.14382582708704916, 46.70000000109248361 ) ) ;
#14462=DIRECTION ( 'NONE',  ( 2.602085213965211135E-16, -1.000000000000000000, 0.000000000000000000 ) ) ;
#14464=CARTESIAN_POINT ( 'NONE',  ( -1.461580736456473462, 62.53841926354353120, 47.45000000109246230 ) ) ;
#14472=FACE_OUTER_BOUND ( 'NONE', #18625, .T. ) ;
#14473=CARTESIAN_POINT ( 'NONE',  ( 32.50000000000000000, 47.00000000000000711, -35.00000000000000000 ) ) ;
#14477=( LENGTH_UNIT ( ) NAMED_UNIT ( * ) SI_UNIT ( .MILLI., .METRE. ) );
#14485=DIRECTION ( 'NONE',  ( 1.000000000000000000, 0.000000000000000000, -0.000000000000000000 ) ) ;
#14493=DIRECTION ( 'NONE',  ( 0.000000000000000000, 0.000000000000000000, 1.000000000000000000 ) ) ;
#14496=DIRECTION ( 'NONE',  ( 0.000000000000000000, 9.912705577010328508E-16, 1.000000000000000000 ) ) ;
#14503=ADVANCED_FACE ( 'NONE', ( #1451 ), #18220, .F. ) ;
#14508=CARTESIAN_POINT ( 'NONE',  ( 1.035533905932739751, 61.50000000000000000, 45.45000000000000995 ) ) ;
#14512=CARTESIAN_POINT ( 'NONE',  ( -1.767766952966370209, 65.76776695296638309, 49.09999999999999432 ) ) ;
#14518=CARTESIAN_POINT ( 'NONE',  ( -2.500000000000011102, 62.96446609406727646, 47.75000000218493312 ) ) ;
#14530=CARTESIAN_POINT ( 'NONE',  ( -0.8561741729129461742, 66.06698729999999387, 47.80000000109247082 ) ) ;
#14534=EDGE_LOOP ( 'NONE', ( #1912, #7726, #5186, #8998 ) ) ;
#14540=LINE ( 'NONE', #1113, #11525 ) ;
#14544=CARTESIAN_POINT ( 'NONE',  ( -1.530808498934192803E-16, 66.50000000000000000, 47.39999999999999858 ) ) ;
#14546=DIRECTION ( 'NONE',  ( 0.000000000000000000, 0.000000000000000000, 1.000000000000000000 ) ) ;
#14557=CARTESIAN_POINT ( 'NONE',  ( 3.796994071234847710E-16, 61.93301269999999903, 48.35000000109246798 ) ) ;
#14584=DIRECTION ( 'NONE',  ( 1.000000000000000000, -0.000000000000000000, 0.000000000000000000 ) ) ;
#14587=CARTESIAN_POINT ( 'NONE',  ( 2.499999999999996891, 62.96446609406726225, 47.14999999999999147 ) ) ;
#14599=CARTESIAN_POINT ( 'NONE',  ( -1.767766952966369765, 62.23223304703363112, 47.00000000218494733 ) ) ;
#14602=ORIENTED_EDGE ( 'NONE', *, *, #19355, .T. ) ;
#14603=ORIENTED_EDGE ( 'NONE', *, *, #17950, .F. ) ;
#14613=CARTESIAN_POINT ( 'NONE',  ( 1.035533905932738197, 66.50000000000000000, 48.94999999999999574 ) ) ;
#14625=EDGE_CURVE ( 'NONE', #15781, #14815, #8021, .T. ) ;
#14633=ORIENTED_EDGE ( 'NONE', *, *, #18776, .F. ) ;
#14641=CARTESIAN_POINT ( 'NONE',  ( -1.035533905932738641, 66.50000000000000000, 46.64999999999999147 ) ) ;
#14647=EDGE_CURVE ( 'NONE', #13230, #13992, #6450, .T. ) ;
#14654=CARTESIAN_POINT ( 'NONE',  ( -0.8561741729129461742, 66.06698729999999387, 48.80000000109247082 ) ) ;
#14670=EDGE_LOOP ( 'NONE', ( #73, #19190 ) ) ;
#14673=ORIENTED_EDGE ( 'NONE', *, *, #14452, .T. ) ;
#14676=CIRCLE ( 'NONE', #7806, 2.499999999999998668 ) ;
#14709=DIRECTION ( 'NONE',  ( 0.000000000000000000, 0.000000000000000000, -1.000000000000000000 ) ) ;
#14716=VECTOR ( 'NONE', #13822, 1000.000000000000000 ) ;
#14730=CARTESIAN_POINT ( 'NONE',  ( 2.066987300000001415, 64.00000000000000000, 45.95000000109246940 ) ) ;
#14742=CARTESIAN_POINT ( 'NONE',  ( 1.767766952966369987, 65.76776695296638309, 47.29999999999999716 ) ) ;
#14743=CARTESIAN_POINT ( 'NONE',  ( 3.796994071234847710E-16, 61.93301269999999903, 48.35000000109246798 ) ) ;
#14749=AXIS2_PLACEMENT_3D ( 'NONE', #3563, #808, #13952 ) ;
#14752=EDGE_CURVE ( 'NONE', #7844, #6260, #13888, .T. ) ;
#14756=CARTESIAN_POINT ( 'NONE',  ( -1.767766952966370209, 65.76776695296638309, 47.60000000218494165 ) ) ;
#14757=EDGE_CURVE ( 'NONE', #16538, #297, #1252, .T. ) ;
#14760=CARTESIAN_POINT ( 'NONE',  ( -1.265664690411616068E-16, 66.06698730000000808, 48.75000000109246656 ) ) ;
#14766=CARTESIAN_POINT ( 'NONE',  ( 0.000000000000000000, 0.000000000000000000, 30.00000000000000000 ) ) ;
#14779=DIRECTION ( 'NONE',  ( 1.000000000000000000, 0.000000000000000000, -0.000000000000000000 ) ) ;
#14781=VERTEX_POINT ( 'NONE', #8426 ) ;
#14790=CARTESIAN_POINT ( 'NONE',  ( 1.767766952966370653, 62.23223304703363112, 47.09999999999999432 ) ) ;
#14806=CARTESIAN_POINT ( 'NONE',  ( 3.999999999999998224, 67.00000000000000000, 30.00000000000000000 ) ) ;
#14815=VERTEX_POINT ( 'NONE', #4211 ) ;
#14837=CARTESIAN_POINT ( 'NONE',  ( 0.000000000000000000, 64.00000000000000000, 49.99999999999999289 ) ) ;
#14842=CARTESIAN_POINT ( 'NONE',  ( -2.500000000000000888, 62.96446609406726935, 46.84999999999998721 ) ) ;
#14843=CARTESIAN_POINT ( 'NONE',  ( -1.461580736456473462, 62.53841926354353120, 48.25000000109246656 ) ) ;
#14852=CARTESIAN_POINT ( 'NONE',  ( -2.500000000000001776, 64.00000000000000000, 47.70000000218494307 ) ) ;
#14854=CARTESIAN_POINT ( 'NONE',  ( -1.461580736456473906, 65.46158073645646880, 46.45000000109246940 ) ) ;
#14865=CARTESIAN_POINT ( 'NONE',  ( -2.283493650000001818, 64.00000000000000000, 49.87500000054622973 ) ) ;
#14881=CARTESIAN_POINT ( 'NONE',  ( -2.066987300000001415, 63.14382582708705627, 48.80000000109247082 ) ) ;
#14883=ORIENTED_EDGE ( 'NONE', *, *, #12825, .T. ) ;
#14885=( BOUNDED_CURVE ( )  B_SPLINE_CURVE ( 2, ( #849, #15664, #4082, #2235, #5372, #11615, #2412, #2508, #9855 ),
 .UNSPECIFIED., .F., .F. ) 
 B_SPLINE_CURVE_WITH_KNOTS ( ( 3, 2, 2, 2, 3 ),
 ( 0.3571428571428572618, 0.3750000000000000555, 0.3928571428571429047, 0.4107142857142856984, 0.4285714285714284921 ),
 .UNSPECIFIED. ) 
 CURVE ( )  GEOMETRIC_REPRESENTATION_ITEM ( )  RATIONAL_B_SPLINE_CURVE ( ( 0.9999999999999995559, 0.9238795325112871826, 1.000000000000000000, 0.9238795325112867385, 1.000000000000000000, 0.9238795325112867385, 1.000000000000000000, 0.9238795325112869605, 0.9999999999999997780 ) ) 
 REPRESENTATION_ITEM ( '' )  );
#14889=LINE ( 'NONE', #12035, #13760 ) ;
#14900=CARTESIAN_POINT ( 'NONE',  ( 32.50000000000000000, 47.00000000000000711, -32.50000000000000000 ) ) ;
#14920=CARTESIAN_POINT ( 'NONE',  ( 2.500000000000001776, 64.00000000000000000, 45.70000000218494307 ) ) ;
#14921=SHAPE_DEFINITION_REPRESENTATION ( #19290, #12005 ) ;
#14933=CARTESIAN_POINT ( 'NONE',  ( 2.066987300000001415, 64.00000000000000000, 45.15000000109247225 ) ) ;
#14945=CARTESIAN_POINT ( 'NONE',  ( 2.066987300000001859, 63.14382582708704916, 47.70000000109246940 ) ) ;
#14949=ORIENTED_EDGE ( 'NONE', *, *, #10695, .F. ) ;
#14954=CARTESIAN_POINT ( 'NONE',  ( -2.066987300000001859, 64.85617417291294373, 45.70000000109248361 ) ) ;
#14959=CARTESIAN_POINT ( 'NONE',  ( 2.066987300000001859, 64.85617417291294373, 49.40000000109246514 ) ) ;
#14973=ORIENTED_EDGE ( 'NONE', *, *, #16339, .T. ) ;
#14977=CARTESIAN_POINT ( 'NONE',  ( 2.066987300000001859, 64.85617417291294373, 49.20000000109247651 ) ) ;
#14983=EDGE_LOOP ( 'NONE', ( #11457, #16869, #14673, #15969 ) ) ;
#14984=LINE ( 'NONE', #186, #11219 ) ;
#14990=ORIENTED_EDGE ( 'NONE', *, *, #6035, .T. ) ;
#15012=AXIS2_PLACEMENT_3D ( 'NONE', #16107, #5338, #4049 ) ;
#15018=ADVANCED_FACE ( 'NONE', ( #3496 ), #6537, .F. ) ;
#15028=CARTESIAN_POINT ( 'NONE',  ( -2.066987300000001859, 64.85617417291294373, 45.50000000109247367 ) ) ;
#15034=DIRECTION ( 'NONE',  ( 0.000000000000000000, 0.000000000000000000, -1.000000000000000000 ) ) ;
#15039=CARTESIAN_POINT ( 'NONE',  ( -2.066987300000001415, 64.00000000000000000, 47.35000000109246798 ) ) ;
#15061=CARTESIAN_POINT ( 'NONE',  ( -0.8561741729129461742, 66.06698729999999387, 49.60000000109246798 ) ) ;
#15070=ORIENTED_EDGE ( 'NONE', *, *, #16910, .F. ) ;
#15095=LINE ( 'NONE', #16961, #7703 ) ;
#15105=CARTESIAN_POINT ( 'NONE',  ( -2.066987300000000971, 63.14382582708704916, 48.80000000109247082 ) ) ;
#15113=CARTESIAN_POINT ( 'NONE',  ( -1.530808498934192803E-16, 66.50000000000000000, 46.59999999999999432 ) ) ;
#15118=EDGE_CURVE ( 'NONE', #8404, #1836, #8207, .T. ) ;
#15119=EDGE_CURVE ( 'NONE', #13223, #18899, #6910, .T. ) ;
#15120=CARTESIAN_POINT ( 'NONE',  ( -1.035533905932738641, 66.50000000000000000, 48.24999999999999289 ) ) ;
#15135=EDGE_CURVE ( 'NONE', #5010, #908, #2122, .T. ) ;
#15138=CARTESIAN_POINT ( 'NONE',  ( 2.066987300000001415, 64.00000000000000000, 46.15000000109247225 ) ) ;
#15146=CARTESIAN_POINT ( 'NONE',  ( -1.767766952966369765, 62.23223304703363112, 47.80000000218494449 ) ) ;
#15150=CARTESIAN_POINT ( 'NONE',  ( 0.8561741729129460632, 66.06698729999999387, 46.30000000109247082 ) ) ;
#15158=CARTESIAN_POINT ( 'NONE',  ( -2.066987300000001415, 63.14382582708705627, 46.60000000109246088 ) ) ;
#15159=PLANE ( 'NONE',  #2766 ) ;
#15174=EDGE_CURVE ( 'NONE', #12045, #375, #9837, .T. ) ;
#15178=CARTESIAN_POINT ( 'NONE',  ( -1.461580736456473906, 65.46158073645646880, 48.65000000109247225 ) ) ;
#15192=EDGE_LOOP ( 'NONE', ( #17707, #1148, #14949, #2932 ) ) ;
#15203=CARTESIAN_POINT ( 'NONE',  ( 1.461580736456473906, 62.53841926354353120, 47.45000000109246940 ) ) ;
#15205=ORIENTED_EDGE ( 'NONE', *, *, #10219, .T. ) ;
#15217=CARTESIAN_POINT ( 'NONE',  ( 14.99999999999998579, 52.00000000000000711, 23.99999999999997158 ) ) ;
#15229=FACE_OUTER_BOUND ( 'NONE', #14394, .T. ) ;
#15236=CARTESIAN_POINT ( 'NONE',  ( -0.8561741729129461742, 66.06698730000000808, 44.80000000109246372 ) ) ;
#15238=LINE ( 'NONE', #1806, #457 ) ;
#15243=CARTESIAN_POINT ( 'NONE',  ( -1.530808498934192803E-16, 66.50000000000000000, 45.10000000218494165 ) ) ;
#15252=CYLINDRICAL_SURFACE ( 'NONE', #5911, 2.500000000000001776 ) ;
#15254=CARTESIAN_POINT ( 'NONE',  ( -1.461580736456473906, 65.46158073645646880, 48.85000000109246798 ) ) ;
#15274=VERTEX_POINT ( 'NONE', #6815 ) ;
#15275=PLANE ( 'NONE',  #3456 ) ;
#15290=VERTEX_POINT ( 'NONE', #10028 ) ;
#15295=CARTESIAN_POINT ( 'NONE',  ( 3.796994071234847710E-16, 61.93301269999999903, 48.95000000109246940 ) ) ;
#15300=CARTESIAN_POINT ( 'NONE',  ( -24.00000000000000000, 0.000000000000000000, -50.00000000000000000 ) ) ;
#15304=FACE_OUTER_BOUND ( 'NONE', #4020, .T. ) ;
#15315=EDGE_LOOP ( 'NONE', ( #11442, #11498, #5465, #17510 ) ) ;
#15328=LINE ( 'NONE', #18475, #15661 ) ;
#15339=CARTESIAN_POINT ( 'NONE',  ( -1.767766952966369765, 62.23223304703363112, 46.20000000218494307 ) ) ;
#15348=CARTESIAN_POINT ( 'NONE',  ( 2.500000000000001776, 64.00000000000000000, 45.59999999999999432 ) ) ;
#15349=CARTESIAN_POINT ( 'NONE',  ( -0.8561741729129461742, 66.06698729999999387, 47.20000000109247651 ) ) ;
#15351=CARTESIAN_POINT ( 'NONE',  ( -15.00000000000000000, 50.00000000000000000, 30.00000000000000000 ) ) ;
#15371=CARTESIAN_POINT ( 'NONE',  ( 2.066987300000001415, 64.00000000000000000, 45.95000000109246940 ) ) ;
#15382=VECTOR ( 'NONE', #10635, 1000.000000000000000 ) ;
#15394=EDGE_LOOP ( 'NONE', ( #5584, #19027, #2738, #18749, #5074, #142, #9638, #4686, #18818, #6687, #10447, #17616, #84, #2947, #2741, #715 ) ) ;
#15397=CARTESIAN_POINT ( 'NONE',  ( -1.265664690411616068E-16, 66.06698730000000808, 46.95000000109246940 ) ) ;
#15428=CARTESIAN_POINT ( 'NONE',  ( -10.00000000000000000, 47.00000000000000711, 30.00000000000000000 ) ) ;
#15429=ORIENTED_EDGE ( 'NONE', *, *, #7438, .F. ) ;
#15435=CARTESIAN_POINT ( 'NONE',  ( -2.066987300000001415, 64.00000000000000000, 44.95000000109246940 ) ) ;
#15441=CARTESIAN_POINT ( 'NONE',  ( 1.035533905932738197, 66.50000000000000000, 45.05000000218494449 ) ) ;
#15449=CARTESIAN_POINT ( 'NONE',  ( 0.8561741729129460632, 66.06698729999999387, 47.10000000109246798 ) ) ;
#15450=CARTESIAN_POINT ( 'NONE',  ( 4.592425496802577917E-16, 61.50000000000000000, 49.39999999999999147 ) ) ;
#15464=CARTESIAN_POINT ( 'NONE',  ( -1.461580736456473462, 62.53841926354353120, 44.85000000109246798 ) ) ;
#15469=FACE_OUTER_BOUND ( 'NONE', #5376, .T. ) ;
#15478=DIRECTION ( 'NONE',  ( -0.000000000000000000, 1.000000000000000000, -0.000000000000000000 ) ) ;
#15489=CARTESIAN_POINT ( 'NONE',  ( -1.265664690411616068E-16, 66.06698730000000808, 48.55000000109247082 ) ) ;
#15496=ORIENTED_EDGE ( 'NONE', *, *, #1617, .F. ) ;
#15507=DIRECTION ( 'NONE',  ( -1.000000000000000000, 0.000000000000000000, 0.000000000000000000 ) ) ;
#15510=DIRECTION ( 'NONE',  ( -0.000000000000000000, 0.000000000000000000, 1.000000000000000000 ) ) ;
#15515=EDGE_CURVE ( 'NONE', #7101, #232, #1910, .T. ) ;
#15531=CARTESIAN_POINT ( 'NONE',  ( -32.50000000000000000, 52.00000000000000711, -35.00000000000000000 ) ) ;
#15537=CARTESIAN_POINT ( 'NONE',  ( -1.035533905932738863, 61.50000000000000000, 44.65000000218494591 ) ) ;
#15542=AXIS2_PLACEMENT_3D ( 'NONE', #12168, #121, #13341 ) ;
#15547=CARTESIAN_POINT ( 'NONE',  ( 2.500000000000001776, 64.00000000000000000, 49.60000000000000142 ) ) ;
#15562=CARTESIAN_POINT ( 'NONE',  ( -2.066987300000001415, 64.00000000000000000, 46.35000000109246798 ) ) ;
#15566=CARTESIAN_POINT ( 'NONE',  ( -1.265664690411616068E-16, 66.06698730000000808, 44.55000000109247082 ) ) ;
#15568=CARTESIAN_POINT ( 'NONE',  ( 14.99999999999998579, 52.00000000000000711, 26.99999999999997158 ) ) ;
#15573=CARTESIAN_POINT ( 'NONE',  ( 32.50000000000000000, 52.00000000000000711, -32.50000000000000000 ) ) ;
#15583=CARTESIAN_POINT ( 'NONE',  ( -2.500000000000003997, 65.03553390593273775, 47.55000000000000426 ) ) ;
#15589=VERTEX_POINT ( 'NONE', #1622 ) ;
#15601=EDGE_CURVE ( 'NONE', #12045, #4427, #13015, .T. ) ;
#15603=EDGE_CURVE ( 'NONE', #16897, #16279, #18289, .T. ) ;
#15626=CARTESIAN_POINT ( 'NONE',  ( 2.500000000000001776, 64.00000000000000000, 44.90000000218493881 ) ) ;
#15637=CARTESIAN_POINT ( 'NONE',  ( 1.035533905932738197, 66.50000000000000000, 49.75000000000000000 ) ) ;
#15642=CARTESIAN_POINT ( 'NONE',  ( 2.500000000000001776, 64.00000000000000000, 47.30000000218494449 ) ) ;
#15650=CARTESIAN_POINT ( 'NONE',  ( 2.066987300000001415, 64.85617417291294373, 46.80000000109247082 ) ) ;
#15655=CARTESIAN_POINT ( 'NONE',  ( -2.066987300000001859, 64.85617417291294373, 46.30000000109247082 ) ) ;
#15657=EDGE_CURVE ( 'NONE', #5462, #4687, #12089, .T. ) ;
#15660=CARTESIAN_POINT ( 'NONE',  ( 41.00000000000000000, 47.00000000000000711, -50.00000000000000000 ) ) ;
#15661=VECTOR ( 'NONE', #1907, 1000.000000000000000 ) ;
#15664=CARTESIAN_POINT ( 'NONE',  ( 2.499999999999996891, 62.96446609406726225, 47.94999999999998863 ) ) ;
#15669=VERTEX_POINT ( 'NONE', #4560 ) ;
#15683=ORIENTED_EDGE ( 'NONE', *, *, #4947, .T. ) ;
#15689=ORIENTED_EDGE ( 'NONE', *, *, #16114, .T. ) ;
#15696=LINE ( 'NONE', #2265, #7857 ) ;
#15698=CARTESIAN_POINT ( 'NONE',  ( 2.499999999999992895, 65.03553390593273775, 49.64999999999998437 ) ) ;
#15708=CARTESIAN_POINT ( 'NONE',  ( -1.767766952966370209, 65.76776695296638309, 45.89999999999999858 ) ) ;
#15710=FACE_OUTER_BOUND ( 'NONE', #13583, .T. ) ;
#15727=CARTESIAN_POINT ( 'NONE',  ( 3.999999999999998224, 67.00000000000000000, 30.00000000000000000 ) ) ;
#15731=CARTESIAN_POINT ( 'NONE',  ( 1.461580736456473684, 65.46158073645646880, 49.25000000109246656 ) ) ;
#15740=CARTESIAN_POINT ( 'NONE',  ( 2.066987300000001859, 64.85617417291294373, 45.40000000109246514 ) ) ;
#15744=CARTESIAN_POINT ( 'NONE',  ( 32.50000000000000000, 52.00000000000000711, 17.49999999999999645 ) ) ;
#15748=CARTESIAN_POINT ( 'NONE',  ( -0.8561741729129466183, 61.93301270000000613, 45.70000000109248361 ) ) ;
#15752=EDGE_CURVE ( 'NONE', #3686, #18580, #9729, .T. ) ;
#15754=CARTESIAN_POINT ( 'NONE',  ( -2.066987300000001415, 63.14382582708705627, 48.00000000109246656 ) ) ;
#15758=CARTESIAN_POINT ( 'NONE',  ( 1.035533905932739751, 61.50000000000000000, 45.55000000218493739 ) ) ;
#15760=CARTESIAN_POINT ( 'NONE',  ( -3.999999999999996447, 47.00000000000000711, 34.99999999999999289 ) ) ;
#15762=DIRECTION ( 'NONE',  ( 0.000000000000000000, 0.000000000000000000, 1.000000000000000000 ) ) ;
#15764=ADVANCED_FACE ( 'NONE', ( #18859 ), #12858, .F. ) ;
#15780=DIRECTION ( 'NONE',  ( 0.000000000000000000, 0.000000000000000000, -1.000000000000000000 ) ) ;
#15781=VERTEX_POINT ( 'NONE', #17287 ) ;
#15791=EDGE_CURVE ( 'NONE', #13516, #3717, #7992, .T. ) ;
#15792=ORIENTED_EDGE ( 'NONE', *, *, #18759, .T. ) ;
#15793=ORIENTED_EDGE ( 'NONE', *, *, #14752, .T. ) ;
#15801=DIRECTION ( 'NONE',  ( 1.000000000000000000, -0.000000000000000000, 0.000000000000000000 ) ) ;
#15806=CARTESIAN_POINT ( 'NONE',  ( -14.99999999999999645, 47.00000000000000711, 23.99999999999997868 ) ) ;
#15808=AXIS2_PLACEMENT_3D ( 'NONE', #8197, #5250, #6712 ) ;
#15810=CARTESIAN_POINT ( 'NONE',  ( -15.00000000000000000, 49.99999999999997158, -4.956352788505161414E-14 ) ) ;
#15817=AXIS2_PLACEMENT_3D ( 'NONE', #2915, #4594, #17818 ) ;
#15818=CARTESIAN_POINT ( 'NONE',  ( -0.8561741729129465073, 61.93301270000000613, 48.10000000109246798 ) ) ;
#15826=CARTESIAN_POINT ( 'NONE',  ( 1.461580736456473906, 62.53841926354353120, 46.05000000109246372 ) ) ;
#15827=CARTESIAN_POINT ( 'NONE',  ( -2.500000000000001776, 64.00000000000000000, 49.19999999999999574 ) ) ;
#15838=CARTESIAN_POINT ( 'NONE',  ( 1.461580736456473684, 65.46158073645646880, 46.05000000109246372 ) ) ;
#15844=CARTESIAN_POINT ( 'NONE',  ( 2.066987300000001415, 64.00000000000000000, 48.55000000109247082 ) ) ;
#15858=ORIENTED_EDGE ( 'NONE', *, *, #18595, .T. ) ;
#15892=CARTESIAN_POINT ( 'NONE',  ( -1.035533905932738641, 66.50000000000000000, 49.04999999999999716 ) ) ;
#15910=CARTESIAN_POINT ( 'NONE',  ( 1.461580736456473684, 65.46158073645646880, 47.65000000109247225 ) ) ;
#15914=FACE_BOUND ( 'NONE', #12957, .T. ) ;
#15922=CARTESIAN_POINT ( 'NONE',  ( -2.066987300000001859, 64.85617417291294373, 44.90000000109247225 ) ) ;
#15923=CARTESIAN_POINT ( 'NONE',  ( 0.8561741729129460632, 66.06698730000000808, 48.70000000109247651 ) ) ;
#15926=DIRECTION ( 'NONE',  ( 2.602085213965211135E-16, -1.000000000000000000, 0.000000000000000000 ) ) ;
#15929=CARTESIAN_POINT ( 'NONE',  ( 2.066987300000001859, 63.14382582708704916, 45.90000000109247225 ) ) ;
#15934=CARTESIAN_POINT ( 'NONE',  ( -2.066987300000001415, 64.00000000000000000, 44.75000000109247367 ) ) ;
#15937=DIRECTION ( 'NONE',  ( 0.000000000000000000, -1.000000000000000000, 0.000000000000000000 ) ) ;
#15942=EDGE_CURVE ( 'NONE', #15290, #10386, #16669, .T. ) ;
#15969=ORIENTED_EDGE ( 'NONE', *, *, #6076, .F. ) ;
#15978=AXIS2_PLACEMENT_3D ( 'NONE', #9527, #2090, #14039 ) ;
#15990=EDGE_CURVE ( 'NONE', #14781, #3001, #14028, .T. ) ;
#15992=ORIENTED_EDGE ( 'NONE', *, *, #7601, .T. ) ;
#15996=CARTESIAN_POINT ( 'NONE',  ( -1.035533905932738641, 66.50000000000000000, 46.75000000218494733 ) ) ;
#16001=CARTESIAN_POINT ( 'NONE',  ( 4.592425496802577917E-16, 61.50000000000000000, 47.90000000218494591 ) ) ;
#16015=CARTESIAN_POINT ( 'NONE',  ( -2.066987300000001415, 64.00000000000000000, 47.95000000109246940 ) ) ;
#16025=CARTESIAN_POINT ( 'NONE',  ( 2.500000000000001776, 65.03553390593273775, 47.24999999999999289 ) ) ;
#16033=CARTESIAN_POINT ( 'NONE',  ( 1.461580736456473906, 62.53841926354353120, 45.05000000109246372 ) ) ;
#16037=CARTESIAN_POINT ( 'NONE',  ( -2.066987300000001859, 64.85617417291294373, 49.70000000109248361 ) ) ;
#16049=ORIENTED_EDGE ( 'NONE', *, *, #4371, .T. ) ;
#16059=ORIENTED_EDGE ( 'NONE', *, *, #8414, .F. ) ;
#16061=VERTEX_POINT ( 'NONE', #14029 ) ;
#16089=EDGE_CURVE ( 'NONE', #14781, #9140, #13027, .T. ) ;
#16097=ORIENTED_EDGE ( 'NONE', *, *, #9414, .T. ) ;
#16101=CARTESIAN_POINT ( 'NONE',  ( -0.8561741729129461742, 66.06698729999999387, 47.00000000109247367 ) ) ;
#16107=CARTESIAN_POINT ( 'NONE',  ( 0.000000000000000000, 47.00000000000000711, -67.72004514666936359 ) ) ;
#16108=LINE ( 'NONE', #13451, #16254 ) ;
#16114=EDGE_CURVE ( 'NONE', #2938, #9711, #11460, .T. ) ;
#16115=CARTESIAN_POINT ( 'NONE',  ( 1.035533905932738197, 66.50000000000000000, 47.34999999999999432 ) ) ;
#16116=CARTESIAN_POINT ( 'NONE',  ( 1.461580736456473684, 65.46158073645646880, 49.45000000109246940 ) ) ;
#16120=AXIS2_PLACEMENT_3D ( 'NONE', #15806, #14329, #19134 ) ;
#16126=CARTESIAN_POINT ( 'NONE',  ( 1.461580736456473684, 65.46158073645646880, 47.05000000109247082 ) ) ;
#16164=DIRECTION ( 'NONE',  ( -0.000000000000000000, 1.000000000000000000, -0.000000000000000000 ) ) ;
#16169=ORIENTED_EDGE ( 'NONE', *, *, #14048, .T. ) ;
#16179=CARTESIAN_POINT ( 'NONE',  ( -1.035533905932738641, 66.50000000000000000, 44.35000000218494165 ) ) ;
#16193=CYLINDRICAL_SURFACE ( 'NONE', #5839, 2.500000000000001776 ) ;
#16197=CARTESIAN_POINT ( 'NONE',  ( 0.8561741729129472844, 61.93301270000000613, 45.80000000109246372 ) ) ;
#16209=CARTESIAN_POINT ( 'NONE',  ( -2.500000000000000888, 62.96446609406726935, 46.04999999999999005 ) ) ;
#16210=CARTESIAN_POINT ( 'NONE',  ( -2.066987300000001415, 64.85617417291294373, 47.30000000109247082 ) ) ;
#16221=CARTESIAN_POINT ( 'NONE',  ( -1.461580736456473906, 65.46158073645646880, 44.65000000109246514 ) ) ;
#16237=PLANE ( 'NONE',  #3469 ) ;
#16240=EDGE_CURVE ( 'NONE', #5462, #6482, #3026, .T. ) ;
#16254=VECTOR ( 'NONE', #1202, 1000.000000000000000 ) ;
#16278=DIRECTION ( 'NONE',  ( 1.000000000000000000, -0.000000000000000000, 0.000000000000000000 ) ) ;
#16279=VERTEX_POINT ( 'NONE', #4832 ) ;
#16289=PLANE ( 'NONE',  #7077 ) ;
#16295=CARTESIAN_POINT ( 'NONE',  ( 2.066987300000001859, 64.85617417291294373, 45.20000000109248361 ) ) ;
#16307=CARTESIAN_POINT ( 'NONE',  ( -2.500000000000001776, 64.00000000000000000, 45.30000000218493739 ) ) ;
#16311=CARTESIAN_POINT ( 'NONE',  ( -2.500000000000001776, 64.00000000000000000, 46.00000000000000000 ) ) ;
#16312=CARTESIAN_POINT ( 'NONE',  ( -0.8561741729129461742, 66.06698730000000808, 46.40000000109247225 ) ) ;
#16325=CARTESIAN_POINT ( 'NONE',  ( -1.035533905932738641, 66.50000000000000000, 47.55000000218494449 ) ) ;
#16336=DIRECTION ( 'NONE',  ( -0.000000000000000000, 0.000000000000000000, 1.000000000000000000 ) ) ;
#16339=EDGE_CURVE ( 'NONE', #19196, #3058, #4531, .T. ) ;
#16350=DIRECTION ( 'NONE',  ( 0.000000000000000000, -0.000000000000000000, -1.000000000000000000 ) ) ;
#16372=DIRECTION ( 'NONE',  ( -0.000000000000000000, -0.000000000000000000, -1.000000000000000000 ) ) ;
#16381=CARTESIAN_POINT ( 'NONE',  ( -1.530808498934192803E-16, 66.50000000000000000, 44.30000000218494449 ) ) ;
#16382=VERTEX_POINT ( 'NONE', #5849 ) ;
#16395=ORIENTED_EDGE ( 'NONE', *, *, #18595, .F. ) ;
#16403=FACE_OUTER_BOUND ( 'NONE', #11334, .T. ) ;
#16405=CARTESIAN_POINT ( 'NONE',  ( -1.530808498934192803E-16, 66.50000000000000000, 45.10000000218494165 ) ) ;
#16406=FACE_BOUND ( 'NONE', #4845, .T. ) ;
#16410=CARTESIAN_POINT ( 'NONE',  ( 0.8561741729129460632, 66.06698730000000808, 46.30000000109247082 ) ) ;
#16420=CARTESIAN_POINT ( 'NONE',  ( 3.796994071234847710E-16, 61.93301269999999903, 46.75000000109246656 ) ) ;
#16426=CARTESIAN_POINT ( 'NONE',  ( 0.8561741729129460632, 66.06698729999999387, 49.50000000109246656 ) ) ;
#16429=DIRECTION ( 'NONE',  ( 1.000000000000000000, 0.000000000000000000, 0.000000000000000000 ) ) ;
#16441=VERTEX_POINT ( 'NONE', #12208 ) ;
#16445=VECTOR ( 'NONE', #2831, 1000.000000000000000 ) ;
#16462=VECTOR ( 'NONE', #3313, 1000.000000000000000 ) ;
#16481=VECTOR ( 'NONE', #12503, 1000.000000000000000 ) ;
#16499=EDGE_CURVE ( 'NONE', #16061, #10386, #646, .T. ) ;
#16500=CARTESIAN_POINT ( 'NONE',  ( -1.265664690411616068E-16, 66.06698730000000808, 45.35000000109246798 ) ) ;
#16507=CARTESIAN_POINT ( 'NONE',  ( 41.00000000000000000, 47.00000000000000711, 30.00000000000000000 ) ) ;
#16508=FACE_OUTER_BOUND ( 'NONE', #11428, .T. ) ;
#16511=CARTESIAN_POINT ( 'NONE',  ( -2.066987300000000971, 63.14382582708704916, 48.20000000109247651 ) ) ;
#16519=CARTESIAN_POINT ( 'NONE',  ( 2.500000000000001776, 64.00000000000000000, 48.10000000218494165 ) ) ;
#16521=CARTESIAN_POINT ( 'NONE',  ( -2.066987300000001415, 63.14382582708705627, 45.80000000109246372 ) ) ;
#16526=CARTESIAN_POINT ( 'NONE',  ( 32.50000000000000000, 47.00000000000000711, 15.00000000000000000 ) ) ;
#16534=VERTEX_POINT ( 'NONE', #5160 ) ;
#16538=VERTEX_POINT ( 'NONE', #15642 ) ;
#16561=ORIENTED_EDGE ( 'NONE', *, *, #19355, .F. ) ;
#16567=ORIENTED_EDGE ( 'NONE', *, *, #1267, .F. ) ;
#16570=ADVANCED_FACE ( 'NONE', ( #7915 ), #454, .F. ) ;
#16571=CARTESIAN_POINT ( 'NONE',  ( -2.066987300000000971, 63.14382582708704916, 48.00000000109246656 ) ) ;
#16576=CARTESIAN_POINT ( 'NONE',  ( 4.000000000000000888, 47.00000000000000711, 30.00000000000000000 ) ) ;
#16584=DIRECTION ( 'NONE',  ( 1.000000000000000000, 0.000000000000000000, 0.000000000000000000 ) ) ;
#16587=CARTESIAN_POINT ( 'NONE',  ( 2.499999999999992895, 65.03553390593275196, 48.15000000218495302 ) ) ;
#16591=LINE ( 'NONE', #19238, #9896 ) ;
#16592=EDGE_CURVE ( 'NONE', #3058, #6376, #11259, .T. ) ;
#16610=CARTESIAN_POINT ( 'NONE',  ( -2.066987300000001415, 64.00000000000000000, 48.15000000109247225 ) ) ;
#16615=DIRECTION ( 'NONE',  ( 0.000000000000000000, 0.000000000000000000, 1.000000000000000000 ) ) ;
#16622=CARTESIAN_POINT ( 'NONE',  ( 2.500000000000001776, 64.00000000000000000, 48.90000000218494591 ) ) ;
#16625=CARTESIAN_POINT ( 'NONE',  ( 0.8561741729129472844, 61.93301270000000613, 46.80000000109246372 ) ) ;
#16630=CARTESIAN_POINT ( 'NONE',  ( 2.500000000000001776, 65.03553390593273775, 45.64999999999999858 ) ) ;
#16632=CARTESIAN_POINT ( 'NONE',  ( -0.8561741729129465073, 61.93301270000000613, 48.30000000109247082 ) ) ;
#16633=FACE_OUTER_BOUND ( 'NONE', #19030, .T. ) ;
#16636=EDGE_CURVE ( 'NONE', #5403, #18922, #6908, .T. ) ;
#16638=DIRECTION ( 'NONE',  ( -0.000000000000000000, 1.000000000000000000, -0.000000000000000000 ) ) ;
#16650=DIRECTION ( 'NONE',  ( -0.000000000000000000, 0.000000000000000000, 1.000000000000000000 ) ) ;
#16669=( BOUNDED_CURVE ( )  B_SPLINE_CURVE ( 2, ( #1787, #220, #3054, #15120, #13337, #5902, #13540, #10397, #4834 ),
 .UNSPECIFIED., .F., .F. ) 
 B_SPLINE_CURVE_WITH_KNOTS ( ( 3, 2, 2, 2, 3 ),
 ( 0.2857142857142853098, 0.3035714285714282701, 0.3214285714285712858, 0.3392857142857143016, 0.3571428571428572618 ),
 .UNSPECIFIED. ) 
 CURVE ( )  GEOMETRIC_REPRESENTATION_ITEM ( )  RATIONAL_B_SPLINE_CURVE ( ( 1.000000000000001554, 0.9238795325112850731, 1.000000000000000000, 0.9238795325112867385, 1.000000000000000000, 0.9238795325112867385, 1.000000000000000000, 0.9238795325112862944, 1.000000000000000444 ) ) 
 REPRESENTATION_ITEM ( '' )  );
#16685=CARTESIAN_POINT ( 'NONE',  ( -1.767766952966370209, 65.76776695296638309, 46.69999999999999574 ) ) ;
#16718=CARTESIAN_POINT ( 'NONE',  ( -1.530808498934192803E-16, 66.50000000000000000, 46.70000000218494307 ) ) ;
#16720=CARTESIAN_POINT ( 'NONE',  ( 1.461580736456473684, 65.46158073645646880, 46.25000000109246656 ) ) ;
#16724=CARTESIAN_POINT ( 'NONE',  ( -2.500000000000001776, 64.00000000000000000, 46.79999999999999716 ) ) ;
#16727=CARTESIAN_POINT ( 'NONE',  ( -1.530808498934192803E-16, 66.50000000000000000, 45.79999999999999005 ) ) ;
#16729=CARTESIAN_POINT ( 'NONE',  ( 1.461580736456473906, 62.53841926354353120, 48.45000000109246940 ) ) ;
#16730=LINE ( 'NONE', #12308, #6226 ) ;
#16745=CARTESIAN_POINT ( 'NONE',  ( -0.8561741729129461742, 66.06698729999999387, 48.60000000109246798 ) ) ;
#16770=CARTESIAN_POINT ( 'NONE',  ( 1.461580736456473684, 65.46158073645646880, 48.45000000109247651 ) ) ;
#16771=CARTESIAN_POINT ( 'NONE',  ( 2.500000000000001776, 64.00000000000000000, 48.90000000218494591 ) ) ;
#16772=EDGE_CURVE ( 'NONE', #9140, #14781, #19235, .T. ) ;
#16775=EDGE_LOOP ( 'NONE', ( #10201, #16059, #15205, #11950 ) ) ;
#16779=DIRECTION ( 'NONE',  ( -0.000000000000000000, -0.000000000000000000, -1.000000000000000000 ) ) ;
#16804=CARTESIAN_POINT ( 'NONE',  ( 41.00000000000000000, 47.00000000000000711, 18.00000000000000000 ) ) ;
#16806=CARTESIAN_POINT ( 'NONE',  ( -1.461580736456473906, 65.46158073645646880, 44.85000000109246798 ) ) ;
#16816=CARTESIAN_POINT ( 'NONE',  ( -1.035533905932738863, 61.50000000000000000, 45.45000000218495018 ) ) ;
#16819=VECTOR ( 'NONE', #13023, 1000.000000000000000 ) ;
#16825=DIRECTION ( 'NONE',  ( -1.000000000000000000, 0.000000000000000000, 0.000000000000000000 ) ) ;
#16827=CARTESIAN_POINT ( 'NONE',  ( -2.066987300000001415, 63.14382582708705627, 47.40000000109247225 ) ) ;
#16828=CARTESIAN_POINT ( 'NONE',  ( -2.500000000000001776, 64.00000000000000000, 45.19999999999999574 ) ) ;
#16844=CARTESIAN_POINT ( 'NONE',  ( -1.461580736456473462, 62.53841926354353120, 47.25000000109247367 ) ) ;
#16846=EDGE_LOOP ( 'NONE', ( #8721, #8135, #18078, #10275 ) ) ;
#16853=LINE ( 'NONE', #13997, #18469 ) ;
#16860=ORIENTED_EDGE ( 'NONE', *, *, #17646, .T. ) ;
#16867=CARTESIAN_POINT ( 'NONE',  ( -2.066987300000001415, 64.85617417291294373, 47.10000000109246798 ) ) ;
#16869=ORIENTED_EDGE ( 'NONE', *, *, #2594, .T. ) ;
#16881=CARTESIAN_POINT ( 'NONE',  ( 2.500000000000007550, 65.03553390593272354, 48.95000000218495018 ) ) ;
#16892=VECTOR ( 'NONE', #9198, 1000.000000000000000 ) ;
#16897=VERTEX_POINT ( 'NONE', #4854 ) ;
#16899=CARTESIAN_POINT ( 'NONE',  ( -2.499999999999996003, 62.96446609406726225, 46.04999999999999005 ) ) ;
#16900=( BOUNDED_CURVE ( )  B_SPLINE_CURVE ( 2, ( #19036, #12601, #1091, #7071, #5606, #9652, #18063, #16587, #7769 ),
 .UNSPECIFIED., .F., .F. ) 
 B_SPLINE_CURVE_WITH_KNOTS ( ( 3, 2, 2, 2, 3 ),
 ( 0.1428571428571428215, 0.1607142857142856429, 0.1785714285714284644, 0.1964285714285712858, 0.2142857142857140795 ),
 .UNSPECIFIED. ) 
 CURVE ( )  GEOMETRIC_REPRESENTATION_ITEM ( )  RATIONAL_B_SPLINE_CURVE ( ( 1.000000000000000222, 0.9238795325112866275, 1.000000000000000000, 0.9238795325112867385, 1.000000000000000000, 0.9238795325112867385, 1.000000000000000000, 0.9238795325112875156, 0.9999999999999992228 ) ) 
 REPRESENTATION_ITEM ( '' )  );
#16910=EDGE_CURVE ( 'NONE', #18801, #4943, #8899, .T. ) ;
#16914=CARTESIAN_POINT ( 'NONE',  ( 2.500000000000002220, 62.96446609406726935, 45.65000000218494591 ) ) ;
#16924=CARTESIAN_POINT ( 'NONE',  ( 14.99999999999998579, 47.00000000000000711, 23.99999999999997158 ) ) ;
#16926=CARTESIAN_POINT ( 'NONE',  ( 2.066987300000001415, 64.00000000000000000, 47.75000000109246656 ) ) ;
#16930=DIRECTION ( 'NONE',  ( 0.000000000000000000, 0.000000000000000000, -1.000000000000000000 ) ) ;
#16939=CIRCLE ( 'NONE', #8470, 2.499999999999998668 ) ;
#16941=ORIENTED_EDGE ( 'NONE', *, *, #7586, .F. ) ;
#16946=CARTESIAN_POINT ( 'NONE',  ( 0.8561741729129472844, 61.93301270000000613, 45.00000000109246656 ) ) ;
#16949=ORIENTED_EDGE ( 'NONE', *, *, #5566, .F. ) ;
#16950=CARTESIAN_POINT ( 'NONE',  ( 14.99999999999998579, 73.00000000000001421, 23.99999999999997158 ) ) ;
#16961=CARTESIAN_POINT ( 'NONE',  ( -32.50000000000000000, 52.00000000000000711, -37.50000000000000711 ) ) ;
#16963=ORIENTED_EDGE ( 'NONE', *, *, #1576, .F. ) ;
#16979=CARTESIAN_POINT ( 'NONE',  ( -32.50000000000000000, 52.00000000000000711, 15.00000000000000000 ) ) ;
#16980=EDGE_CURVE ( 'NONE', #232, #17355, #15238, .T. ) ;
#16989=VECTOR ( 'NONE', #11435, 1000.000000000000000 ) ;
#17004=CARTESIAN_POINT ( 'NONE',  ( 1.035533905932739751, 61.50000000000000000, 46.24999999999999289 ) ) ;
#17014=CARTESIAN_POINT ( 'NONE',  ( -2.500000000000000888, 62.96446609406726935, 44.55000000218495870 ) ) ;
#17025=CARTESIAN_POINT ( 'NONE',  ( -0.8561741729129461742, 66.06698729999999387, 48.80000000109247082 ) ) ;
#17039=CARTESIAN_POINT ( 'NONE',  ( -2.066987300000001859, 64.85617417291294373, 47.10000000109246798 ) ) ;
#17043=DIRECTION ( 'NONE',  ( -0.000000000000000000, 1.000000000000000000, -0.000000000000000000 ) ) ;
#17045=DIRECTION ( 'NONE',  ( -1.000000000000000000, -0.000000000000000000, -0.000000000000000000 ) ) ;
#17070=ORIENTED_EDGE ( 'NONE', *, *, #2528, .T. ) ;
#17072=CARTESIAN_POINT ( 'NONE',  ( 0.000000000000000000, 64.00000000000000000, 49.99999999999999289 ) ) ;
#17078=CARTESIAN_POINT ( 'NONE',  ( 1.767766952966369987, 65.76776695296638309, 49.69999999999999574 ) ) ;
#17096=CYLINDRICAL_SURFACE ( 'NONE', #14749, 2.500000000000001776 ) ;
#17106=CARTESIAN_POINT ( 'NONE',  ( -2.500000000000001776, 65.03553390593273775, 45.25000000218494733 ) ) ;
#17116=CARTESIAN_POINT ( 'NONE',  ( 0.8561741729129472844, 61.93301270000000613, 46.00000000109245946 ) ) ;
#17122=EDGE_LOOP ( 'NONE', ( #4189, #969, #1080, #19114, #10720, #13121, #9949, #5859 ) ) ;
#17130=CARTESIAN_POINT ( 'NONE',  ( -1.461580736456473462, 62.53841926354353120, 45.65000000109247225 ) ) ;
#17144=( NAMED_UNIT ( * ) PLANE_ANGLE_UNIT ( ) SI_UNIT ( $, .RADIAN. ) );
#17145=VERTEX_POINT ( 'NONE', #10293 ) ;
#17155=ORIENTED_EDGE ( 'NONE', *, *, #9935, .T. ) ;
#17162=CYLINDRICAL_SURFACE ( 'NONE', #50, 2.500000000000001776 ) ;
#17169=DIRECTION ( 'NONE',  ( 0.000000000000000000, 0.000000000000000000, 1.000000000000000000 ) ) ;
#17201=CARTESIAN_POINT ( 'NONE',  ( -2.066987300000001859, 64.85617417291294373, 47.90000000109247225 ) ) ;
#17203=LINE ( 'NONE', #4864, #7913 ) ;
#17211=CARTESIAN_POINT ( 'NONE',  ( -2.500000000000001776, 64.00000000000000000, 49.99999999999999289 ) ) ;
#17220=CARTESIAN_POINT ( 'NONE',  ( -1.461580736456473906, 65.46158073645646880, 46.25000000109247367 ) ) ;
#17225=CARTESIAN_POINT ( 'NONE',  ( -0.8561741729129461742, 66.06698729999999387, 45.40000000109246514 ) ) ;
#17232=DIRECTION ( 'NONE',  ( -1.000000000000000000, 0.000000000000000000, 0.000000000000000000 ) ) ;
#17247=LINE ( 'NONE', #9960, #18486 ) ;
#17259=VECTOR ( 'NONE', #4025, 1000.000000000000000 ) ;
#17269=CARTESIAN_POINT ( 'NONE',  ( -2.500000000000001776, 64.00000000000000000, 49.99999999999999289 ) ) ;
#17287=CARTESIAN_POINT ( 'NONE',  ( -15.00000000000000000, 35.00000000000000000, 37.00000000000000000 ) ) ;
#17293=CARTESIAN_POINT ( 'NONE',  ( -1.461580736456473462, 62.53841926354353120, 47.25000000109247367 ) ) ;
#17305=CARTESIAN_POINT ( 'NONE',  ( 2.500000000000001776, 65.03553390593273775, 49.64999999999999147 ) ) ;
#17306=CARTESIAN_POINT ( 'NONE',  ( 2.066987300000001859, 63.14382582708704916, 49.30000000109246372 ) ) ;
#17312=CARTESIAN_POINT ( 'NONE',  ( 1.461580736456473906, 62.53841926354353120, 45.85000000109246798 ) ) ;
#17316=ADVANCED_FACE ( 'NONE', ( #18364 ), #18267, .T. ) ;
#17317=CARTESIAN_POINT ( 'NONE',  ( -1.461580736456473906, 65.46158073645646880, 48.05000000109247082 ) ) ;
#17335=CARTESIAN_POINT ( 'NONE',  ( 2.500000000000001776, 64.00000000000000000, 47.19999999999999574 ) ) ;
#17355=VERTEX_POINT ( 'NONE', #10696 ) ;
#17371=CARTESIAN_POINT ( 'NONE',  ( 32.50000000000000000, 52.00000000000000711, -35.00000000000000000 ) ) ;
#17378=CARTESIAN_POINT ( 'NONE',  ( -0.8561741729129461742, 66.06698729999999387, 48.60000000109246798 ) ) ;
#17383=CARTESIAN_POINT ( 'NONE',  ( 4.592425496802577917E-16, 61.50000000000000000, 46.30000000218493739 ) ) ;
#17390=CARTESIAN_POINT ( 'NONE',  ( -2.066987300000001415, 64.00000000000000000, 45.75000000109247367 ) ) ;
#17401=CARTESIAN_POINT ( 'NONE',  ( -2.066987300000001415, 64.85617417291294373, 46.30000000109247082 ) ) ;
#17407=CARTESIAN_POINT ( 'NONE',  ( 0.8561741729129472844, 61.93301270000000613, 47.60000000109246798 ) ) ;
#17409=ORIENTED_EDGE ( 'NONE', *, *, #10616, .T. ) ;
#17414=CARTESIAN_POINT ( 'NONE',  ( 0.000000000000000000, 64.00000000000000000, 34.99999999999999289 ) ) ;
#17464=LINE ( 'NONE', #4040, #2683 ) ;
#17469=CARTESIAN_POINT ( 'NONE',  ( 0.8561741729129472844, 61.93301270000000613, 47.40000000109247225 ) ) ;
#17474=FACE_OUTER_BOUND ( 'NONE', #15394, .T. ) ;
#17477=DIRECTION ( 'NONE',  ( 0.000000000000000000, 0.000000000000000000, 1.000000000000000000 ) ) ;
#17480=CARTESIAN_POINT ( 'NONE',  ( -1.461580736456473906, 65.46158073645646880, 44.85000000109246798 ) ) ;
#17483=CARTESIAN_POINT ( 'NONE',  ( -2.499999999999999556, 62.96446609406726225, 48.55000000218494449 ) ) ;
#17490=CARTESIAN_POINT ( 'NONE',  ( 2.066987300000001415, 64.85617417291294373, 45.20000000109248361 ) ) ;
#17496=CARTESIAN_POINT ( 'NONE',  ( 2.066987300000002303, 63.14382582708705627, 47.70000000109247651 ) ) ;
#17499=CARTESIAN_POINT ( 'NONE',  ( -1.767766952966369765, 62.23223304703363112, 45.40000000218494591 ) ) ;
#17510=ORIENTED_EDGE ( 'NONE', *, *, #6867, .F. ) ;
#17513=PRESENTATION_STYLE_ASSIGNMENT (( #2517 ) ) ;
#17528=LINE ( 'NONE', #12732, #10004 ) ;
#17540=DIRECTION ( 'NONE',  ( 0.000000000000000000, 0.000000000000000000, 1.000000000000000000 ) ) ;
#17554=CARTESIAN_POINT ( 'NONE',  ( 1.767766952966369987, 65.76776695296638309, 48.89999999999999858 ) ) ;
#17556=VECTOR ( 'NONE', #11067, 1000.000000000000000 ) ;
#17578=CARTESIAN_POINT ( 'NONE',  ( 1.461580736456473684, 65.46158073645646880, 46.85000000109246798 ) ) ;
#17589=CARTESIAN_POINT ( 'NONE',  ( -2.500000000000001776, 64.00000000000000000, 46.79999999999999716 ) ) ;
#17599=FACE_OUTER_BOUND ( 'NONE', #7322, .T. ) ;
#17601=CARTESIAN_POINT ( 'NONE',  ( 0.8561741729129472844, 61.93301270000000613, 48.40000000109247225 ) ) ;
#17603=CARTESIAN_POINT ( 'NONE',  ( -14.99999999999999645, 47.00000000000000711, 23.99999999999997868 ) ) ;
#17609=LINE ( 'NONE', #14370, #1918 ) ;
#17611=VERTEX_POINT ( 'NONE', #13515 ) ;
#17616=ORIENTED_EDGE ( 'NONE', *, *, #5345, .T. ) ;
#17622=DIRECTION ( 'NONE',  ( 0.000000000000000000, 0.000000000000000000, 1.000000000000000000 ) ) ;
#17623=EDGE_LOOP ( 'NONE', ( #10891, #9802, #12755, #552 ) ) ;
#17626=( BOUNDED_CURVE ( )  B_SPLINE_CURVE ( 2, ( #2921, #14587, #14790, #1358, #19299, #13102, #5868, #13398, #13205 ),
 .UNSPECIFIED., .F., .F. ) 
 B_SPLINE_CURVE_WITH_KNOTS ( ( 3, 2, 2, 2, 3 ),
 ( 0.5000000000000001110, 0.5178571428571430157, 0.5357142857142858094, 0.5535714285714286031, 0.5714285714285713969 ),
 .UNSPECIFIED. ) 
 CURVE ( )  GEOMETRIC_REPRESENTATION_ITEM ( )  RATIONAL_B_SPLINE_CURVE ( ( 0.9999999999999995559, 0.9238795325112871826, 1.000000000000000000, 0.9238795325112867385, 1.000000000000000000, 0.9238795325112867385, 1.000000000000000000, 0.9238795325112867385, 1.000000000000000000 ) ) 
 REPRESENTATION_ITEM ( '' )  );
#17631=CYLINDRICAL_SURFACE ( 'NONE', #18757, 2.500000000000001776 ) ;
#17639=VERTEX_POINT ( 'NONE', #19113 ) ;
#17644=ORIENTED_EDGE ( 'NONE', *, *, #12510, .T. ) ;
#17646=EDGE_CURVE ( 'NONE', #9711, #2938, #18662, .T. ) ;
#17649=VERTEX_POINT ( 'NONE', #1271 ) ;
#17657=CARTESIAN_POINT ( 'NONE',  ( 32.50000000000000000, 47.00000000000000711, 15.00000000000000000 ) ) ;
#17664=DIRECTION ( 'NONE',  ( -1.000000000000000000, 0.000000000000000000, -0.000000000000000000 ) ) ;
#17666=ORIENTED_EDGE ( 'NONE', *, *, #17950, .T. ) ;
#17669=CARTESIAN_POINT ( 'NONE',  ( -1.265664690411616068E-16, 66.06698730000000808, 46.15000000109247225 ) ) ;
#17670=EDGE_CURVE ( 'NONE', #7750, #18471, #17837, .T. ) ;
#17681=CARTESIAN_POINT ( 'NONE',  ( -1.035533905932738641, 66.50000000000000000, 48.24999999999999289 ) ) ;
#17682=CARTESIAN_POINT ( 'NONE',  ( -1.265664690411616068E-16, 66.06698730000000808, 46.35000000109246798 ) ) ;
#17684=DIRECTION ( 'NONE',  ( 1.000000000000000000, 0.000000000000000000, 0.000000000000000000 ) ) ;
#17688=AXIS2_PLACEMENT_3D ( 'NONE', #16804, #1905, #7889 ) ;
#17693=CARTESIAN_POINT ( 'NONE',  ( -2.500000000000001776, 65.03553390593273775, 47.65000000218494591 ) ) ;
#17695=CARTESIAN_POINT ( 'NONE',  ( 1.461580736456473684, 65.46158073645646880, 47.85000000109246798 ) ) ;
#17707=ORIENTED_EDGE ( 'NONE', *, *, #7438, .T. ) ;
#17713=VECTOR ( 'NONE', #3685, 1000.000000000000000 ) ;
#17723=ORIENTED_EDGE ( 'NONE', *, *, #1853, .T. ) ;
#17737=VERTEX_POINT ( 'NONE', #4119 ) ;
#17742=LINE ( 'NONE', #14806, #4608 ) ;
#17744=ORIENTED_EDGE ( 'NONE', *, *, #4850, .F. ) ;
#17750=DIRECTION ( 'NONE',  ( -1.000000000000000000, 0.000000000000000000, 0.000000000000000000 ) ) ;
#17762=CARTESIAN_POINT ( 'NONE',  ( -4.000000000000001776, 67.00000000000000000, 30.00000000000000000 ) ) ;
#17775=ORIENTED_EDGE ( 'NONE', *, *, #2948, .T. ) ;
#17783=CARTESIAN_POINT ( 'NONE',  ( -1.767766952966370209, 65.76776695296638309, 46.69999999999999574 ) ) ;
#17784=CARTESIAN_POINT ( 'NONE',  ( -1.265664690411616068E-16, 66.06698730000000808, 47.15000000109247225 ) ) ;
#17795=CARTESIAN_POINT ( 'NONE',  ( -1.767766952966369765, 62.23223304703363112, 48.60000000218494165 ) ) ;
#17816=ORIENTED_EDGE ( 'NONE', *, *, #6786, .T. ) ;
#17818=DIRECTION ( 'NONE',  ( 0.000000000000000000, 0.000000000000000000, -1.000000000000000000 ) ) ;
#17821=CARTESIAN_POINT ( 'NONE',  ( 1.461580736456473684, 65.46158073645646880, 49.25000000109246656 ) ) ;
#17834=DIRECTION ( 'NONE',  ( -0.000000000000000000, -1.000000000000000000, 0.000000000000000000 ) ) ;
#17837=LINE ( 'NONE', #5777, #16445 ) ;
#17847=EDGE_CURVE ( 'NONE', #18801, #10345, #15095, .T. ) ;
#17861=LINE ( 'NONE', #6097, #19136 ) ;
#17869=CYLINDRICAL_SURFACE ( 'NONE', #2389, 2.500000000000001776 ) ;
#17884=CARTESIAN_POINT ( 'NONE',  ( 2.500000000000002220, 62.96446609406726225, 45.54999999999999005 ) ) ;
#17888=CARTESIAN_POINT ( 'NONE',  ( -1.461580736456473462, 62.53841926354353120, 45.85000000109246798 ) ) ;
#17889=VECTOR ( 'NONE', #7530, 1000.000000000000000 ) ;
#17891=CARTESIAN_POINT ( 'NONE',  ( 0.000000000000000000, 64.00000000000000000, 49.99999999999999289 ) ) ;
#17903=CARTESIAN_POINT ( 'NONE',  ( 1.461580736456473906, 62.53841926354353120, 46.85000000109246798 ) ) ;
#17908=VECTOR ( 'NONE', #3300, 1000.000000000000000 ) ;
#17934=DIRECTION ( 'NONE',  ( -0.000000000000000000, 1.000000000000000000, -0.000000000000000000 ) ) ;
#17938=CARTESIAN_POINT ( 'NONE',  ( 32.50000000000000000, 52.00000000000000711, -35.00000000000000000 ) ) ;
#17949=CARTESIAN_POINT ( 'NONE',  ( -32.50000000000000000, 47.00000000000000711, 15.00000000000000000 ) ) ;
#17950=EDGE_CURVE ( 'NONE', #16534, #19297, #18674, .T. ) ;
#17953=CARTESIAN_POINT ( 'NONE',  ( -2.500000000000001776, 64.00000000000000000, 47.70000000218494307 ) ) ;
#17956=ORIENTED_EDGE ( 'NONE', *, *, #2771, .F. ) ;
#17963=CARTESIAN_POINT ( 'NONE',  ( -1.767766952966370209, 65.76776695296638309, 49.89999999999999147 ) ) ;
#17975=CARTESIAN_POINT ( 'NONE',  ( -15.00000000000000000, 0.000000000000000000, 37.00000000000000000 ) ) ;
#17981=CARTESIAN_POINT ( 'NONE',  ( -2.066987300000001415, 64.85617417291294373, 45.70000000109248361 ) ) ;
#17993=CARTESIAN_POINT ( 'NONE',  ( 2.500000000000001776, 65.03553390593273775, 48.15000000218494591 ) ) ;
#17996=CARTESIAN_POINT ( 'NONE',  ( 3.796994071234847710E-16, 61.93301269999999903, 45.15000000109247225 ) ) ;
#18012=ORIENTED_EDGE ( 'NONE', *, *, #19229, .T. ) ;
#18049=LINE ( 'NONE', #13226, #18476 ) ;
#18054=CARTESIAN_POINT ( 'NONE',  ( -1.767766952966370209, 65.76776695296638309, 47.60000000218494165 ) ) ;
#18063=CARTESIAN_POINT ( 'NONE',  ( 1.767766952966369987, 65.76776695296638309, 48.20000000218494307 ) ) ;
#18075=CARTESIAN_POINT ( 'NONE',  ( -14.99999999999999645, 47.00000000000000711, 20.99999999999998224 ) ) ;
#18078=ORIENTED_EDGE ( 'NONE', *, *, #16980, .T. ) ;
#18083=CARTESIAN_POINT ( 'NONE',  ( -0.8561741729129466183, 61.93301270000000613, 47.50000000109246656 ) ) ;
#18086=UNCERTAINTY_MEASURE_WITH_UNIT (LENGTH_MEASURE( 1.000000000000000082E-05 ), #12843, 'distance_accuracy_value', 'NONE');
#18092=CARTESIAN_POINT ( 'NONE',  ( 1.035533905932738197, 66.50000000000000000, 48.25000000218493312 ) ) ;
#18094=CARTESIAN_POINT ( 'NONE',  ( 0.8561741729129460632, 66.06698729999999387, 45.50000000109247367 ) ) ;
#18099=DIRECTION ( 'NONE',  ( -0.000000000000000000, -0.000000000000000000, -1.000000000000000000 ) ) ;
#18101=CARTESIAN_POINT ( 'NONE',  ( -0.8561741729129461742, 66.06698729999999387, 46.40000000109246514 ) ) ;
#18108=ORIENTED_EDGE ( 'NONE', *, *, #15174, .T. ) ;
#18119=CARTESIAN_POINT ( 'NONE',  ( 1.461580736456473906, 62.53841926354353120, 49.05000000109247082 ) ) ;
#18122=ORIENTED_EDGE ( 'NONE', *, *, #15990, .F. ) ;
#18123=DIRECTION ( 'NONE',  ( 0.000000000000000000, 0.000000000000000000, -1.000000000000000000 ) ) ;
#18125=VERTEX_POINT ( 'NONE', #19377 ) ;
#18128=EDGE_CURVE ( 'NONE', #10014, #3899, #3267, .T. ) ;
#18135=ORIENTED_EDGE ( 'NONE', *, *, #5719, .F. ) ;
#18151=ORIENTED_EDGE ( 'NONE', *, *, #958, .F. ) ;
#18162=( BOUNDED_CURVE ( )  B_SPLINE_CURVE ( 2, ( #13164, #1116, #10117, #18878, #2303, #5630, #16116, #11310, #7097, #17306, #8474, #4059, #3868, #9925, #13061, #12968, #5255, #14349, #5442, #8662, #11397, #15923, #18964, #5535, #11493, #1209, #12085, #13458, #14743, #5732, #14843, #16511, #16610, #137, #1706, #8754, #8858, #1415, #19161, #2777, #7686, #14945, #6120, #1321, #7293, #18083, #11891, #2974, #15039, #16210, #13260, #4557, #17784, #4656, #10316, #19258, #10610, #7389, #1618, #13362, #8952, #9154, #5826, #11691, #13557, #11792, #3176, #16312, #17682, #16410, #11987, #19354, #15138, #10512, #4360, #7483, #4260, #5922, #17888, #4462, #10221, #17981, #10414, #2880, #3073, #1516, #41, #6028, #9052, #7590, #6221, #10907, #12385, #18382, #14047, #6417, #15435, #4951, #16806, #15236, #1999 ),
 .UNSPECIFIED., .F., .F. ) 
 B_SPLINE_CURVE_WITH_KNOTS ( ( 3, 2, 2, 2, 2, 2, 2, 2, 2, 2, 2, 2, 2, 2, 2, 2, 2, 2, 2, 2, 2, 2, 2, 2, 2, 2, 2, 2, 2, 2, 2, 2, 2, 2, 2, 2, 2, 2, 2, 2, 2, 2, 2, 2, 2, 2, 2, 2, 2, 2, 3 ),
 ( 0.000000000000000000, 0.01785714285714285615, 0.03571428571428571230, 0.05357142857142856845, 0.07142857142857142461, 0.08928571428571428770, 0.1071428571428571369, 0.1250000000000000000, 0.1428571428571428492, 0.1607142857142857262, 0.1785714285714285754, 0.1964285714285714246, 0.2142857142857142738, 0.2321428571428571508, 0.2500000000000000000, 0.2678571428571428492, 0.2857142857142856984, 0.3035714285714285476, 0.3214285714285714524, 0.3392857142857143016, 0.3571428571428571508, 0.3750000000000000000, 0.3928571428571428492, 0.4107142857142856984, 0.4285714285714285476, 0.4464285714285714524, 0.4642857142857143016, 0.4821428571428571508, 0.5000000000000000000, 0.5178571428571429047, 0.5357142857142856984, 0.5535714285714286031, 0.5714285714285713969, 0.5892857142857143016, 0.6071428571428570953, 0.6250000000000000000, 0.6428571428571429047, 0.6607142857142856984, 0.6785714285714286031, 0.6964285714285715079, 0.7142857142857143016, 0.7321428571428570953, 0.7500000000000000000, 0.7678571428571429047, 0.7857142857142856984, 0.8035714285714286031, 0.8214285714285713969, 0.8392857142857143016, 0.8571428571428570953, 0.8750000000000000000, 0.8928571428571429047 ),
 .UNSPECIFIED. ) 
 CURVE ( )  GEOMETRIC_REPRESENTATION_ITEM ( )  RATIONAL_B_SPLINE_CURVE ( ( 1.000000000000000000, 0.9238795325112867385, 1.000000000000000000, 0.9238795325112867385, 1.000000000000000000, 0.9238795325112867385, 1.000000000000000000, 0.9238795325112867385, 1.000000000000000000, 0.9238795325112867385, 1.000000000000000000, 0.9238795325112867385, 1.000000000000000000, 0.9238795325112867385, 1.000000000000000000, 0.9238795325112867385, 1.000000000000000000, 0.9238795325112867385, 1.000000000000000000, 0.9238795325112867385, 1.000000000000000000, 0.9238795325112867385, 1.000000000000000000, 0.9238795325112867385, 1.000000000000000000, 0.9238795325112867385, 1.000000000000000000, 0.9238795325112867385, 1.000000000000000000, 0.9238795325112867385, 1.000000000000000000, 0.9238795325112867385, 1.000000000000000000, 0.9238795325112867385, 1.000000000000000000, 0.9238795325112867385, 1.000000000000000000, 0.9238795325112867385, 1.000000000000000000, 0.9238795325112867385, 1.000000000000000000, 0.9238795325112867385, 1.000000000000000000, 0.9238795325112867385, 1.000000000000000000, 0.9238795325112867385, 1.000000000000000000, 0.9238795325112867385, 1.000000000000000000, 0.9238795325112867385, 1.000000000000000000, 0.9238795325112867385, 1.000000000000000000, 0.9238795325112867385, 1.000000000000000000, 0.9238795325112867385, 1.000000000000000000, 0.9238795325112867385, 1.000000000000000000, 0.9238795325112867385, 1.000000000000000000, 0.9238795325112867385, 1.000000000000000000, 0.9238795325112867385, 1.000000000000000000, 0.9238795325112867385, 1.000000000000000000, 0.9238795325112867385, 1.000000000000000000, 0.9238795325112867385, 1.000000000000000000, 0.9238795325112867385, 1.000000000000000000, 0.9238795325112867385, 1.000000000000000000, 0.9238795325112867385, 1.000000000000000000, 0.9238795325112867385, 1.000000000000000000, 0.9238795325112867385, 1.000000000000000000, 0.9238795325112867385, 1.000000000000000000, 0.9238795325112867385, 1.000000000000000000, 0.9238795325112867385, 1.000000000000000000, 0.9238795325112867385, 1.000000000000000000, 0.9238795325112867385, 1.000000000000000000, 0.9238795325112867385, 1.000000000000000000, 0.9238795325112867385, 1.000000000000000000, 0.9238795325112867385, 1.000000000000000000, 0.9238795325112867385, 1.000000000000000000, 0.9238795325112867385, 1.000000000000000000 ) ) 
 REPRESENTATION_ITEM ( '' )  );
#18165=ORIENTED_EDGE ( 'NONE', *, *, #2088, .T. ) ;
#18195=CARTESIAN_POINT ( 'NONE',  ( -1.767766952966370209, 65.76776695296638309, 46.00000000218494733 ) ) ;
#18206=CARTESIAN_POINT ( 'NONE',  ( 1.461580736456473684, 65.46158073645646880, 47.05000000109247082 ) ) ;
#18220=PLANE ( 'NONE',  #14259 ) ;
#18223=CARTESIAN_POINT ( 'NONE',  ( -1.265664690411616068E-16, 66.06698730000000808, 49.35000000109246798 ) ) ;
#18227=AXIS2_PLACEMENT_3D ( 'NONE', #4069, #12977, #9758 ) ;
#18232=LINE ( 'NONE', #10659, #8444 ) ;
#18236=ORIENTED_EDGE ( 'NONE', *, *, #2784, .F. ) ;
#18249=CARTESIAN_POINT ( 'NONE',  ( 2.066987300000001415, 64.00000000000000000, 47.55000000109247082 ) ) ;
#18260=CARTESIAN_POINT ( 'NONE',  ( -3.999999999999999112, 52.00000000000000711, 30.00000000000000000 ) ) ;
#18267=CYLINDRICAL_SURFACE ( 'NONE', #19272, 2.500000000000001776 ) ;
#18280=FACE_OUTER_BOUND ( 'NONE', #7125, .T. ) ;
#18289=LINE ( 'NONE', #240, #5828 ) ;
#18290=ORIENTED_EDGE ( 'NONE', *, *, #15601, .T. ) ;
#18294=CARTESIAN_POINT ( 'NONE',  ( -1.767766952966369765, 62.23223304703363112, 44.60000000218494165 ) ) ;
#18301=CARTESIAN_POINT ( 'NONE',  ( -1.767766952966370209, 65.76776695296638309, 45.89999999999999858 ) ) ;
#18303=CARTESIAN_POINT ( 'NONE',  ( -1.461580736456473462, 62.53841926354353120, 48.25000000109246656 ) ) ;
#18319=CARTESIAN_POINT ( 'NONE',  ( -1.461580736456473906, 65.46158073645646880, 46.25000000109247367 ) ) ;
#18329=CARTESIAN_POINT ( 'NONE',  ( -1.530808498934192803E-16, 66.50000000000000000, 49.99999999999999289 ) ) ;
#18343=CARTESIAN_POINT ( 'NONE',  ( -2.066987300000000971, 63.14382582708704916, 47.20000000109248361 ) ) ;
#18344=CARTESIAN_POINT ( 'NONE',  ( 2.500000000000001776, 64.00000000000000000, 49.60000000000000142 ) ) ;
#18364=FACE_OUTER_BOUND ( 'NONE', #15192, .T. ) ;
#18380=CARTESIAN_POINT ( 'NONE',  ( 2.500000000000001776, 64.00000000000000000, 46.39999999999999858 ) ) ;
#18382=CARTESIAN_POINT ( 'NONE',  ( -0.8561741729129466183, 61.93301270000000613, 45.10000000109246798 ) ) ;
#18390=CARTESIAN_POINT ( 'NONE',  ( -2.500000000000001776, 65.03553390593273775, 46.85000000218494165 ) ) ;
#18402=CARTESIAN_POINT ( 'NONE',  ( 0.8561741729129460632, 66.06698729999999387, 48.70000000109247651 ) ) ;
#18403=CARTESIAN_POINT ( 'NONE',  ( 2.500000000000011102, 62.96446609406727646, 49.54999999999999716 ) ) ;
#18405=DIRECTION ( 'NONE',  ( -0.000000000000000000, -1.000000000000000000, -0.000000000000000000 ) ) ;
#18419=CARTESIAN_POINT ( 'NONE',  ( -0.8561741729129465073, 61.93301270000000613, 45.70000000109248361 ) ) ;
#18430=VERTEX_POINT ( 'NONE', #11477 ) ;
#18431=ORIENTED_EDGE ( 'NONE', *, *, #11049, .T. ) ;
#18432=ORIENTED_EDGE ( 'NONE', *, *, #18890, .T. ) ;
#18434=ORIENTED_EDGE ( 'NONE', *, *, #16636, .F. ) ;
#18435=EDGE_LOOP ( 'NONE', ( #13396, #7635, #5996, #4701 ) ) ;
#18460=DIRECTION ( 'NONE',  ( 0.000000000000000000, -1.000000000000000000, 0.000000000000000000 ) ) ;
#18461=ADVANCED_FACE ( 'NONE', ( #5612 ), #2379, .T. ) ;
#18463=EDGE_CURVE ( 'NONE', #4643, #5010, #17464, .T. ) ;
#18469=VECTOR ( 'NONE', #9385, 1000.000000000000000 ) ;
#18470=CARTESIAN_POINT ( 'NONE',  ( 0.000000000000000000, 47.00000000000000711, 30.00000000000000000 ) ) ;
#18471=VERTEX_POINT ( 'NONE', #5513 ) ;
#18473=LINE ( 'NONE', #6318, #12048 ) ;
#18475=CARTESIAN_POINT ( 'NONE',  ( -2.500000000000001776, 64.00000000000000000, 49.65000000109247225 ) ) ;
#18476=VECTOR ( 'NONE', #13320, 1000.000000000000000 ) ;
#18486=VECTOR ( 'NONE', #14584, 1000.000000000000000 ) ;
#18487=CARTESIAN_POINT ( 'NONE',  ( 2.500000000000002220, 62.96446609406726935, 44.85000000218494165 ) ) ;
#18493=CARTESIAN_POINT ( 'NONE',  ( 32.50000000000000000, 47.00000000000000711, 17.49999999999999645 ) ) ;
#18498=CARTESIAN_POINT ( 'NONE',  ( 2.066987300000002303, 63.14382582708705627, 49.30000000109246372 ) ) ;
#18504=AXIS2_PLACEMENT_3D ( 'NONE', #10548, #11818, #13587 ) ;
#18517=CARTESIAN_POINT ( 'NONE',  ( 1.461580736456473684, 65.46158073645646880, 46.85000000109246798 ) ) ;
#18535=ORIENTED_EDGE ( 'NONE', *, *, #9857, .F. ) ;
#18537=ORIENTED_EDGE ( 'NONE', *, *, #14625, .F. ) ;
#18547=LINE ( 'NONE', #5114, #17556 ) ;
#18548=EDGE_LOOP ( 'NONE', ( #13762, #5088, #10076, #19325 ) ) ;
#18575=AXIS2_PLACEMENT_3D ( 'NONE', #18611, #17043, #5176 ) ;
#18577=CYLINDRICAL_SURFACE ( 'NONE', #362, 2.500000000000002220 ) ;
#18580=VERTEX_POINT ( 'NONE', #905 ) ;
#18582=CARTESIAN_POINT ( 'NONE',  ( -1.035533905932738641, 66.50000000000000000, 45.95000000218494307 ) ) ;
#18584=LINE ( 'NONE', #14162, #8441 ) ;
#18586=CARTESIAN_POINT ( 'NONE',  ( -32.50000000000000000, 47.00000000000000711, 17.49999999999999645 ) ) ;
#18590=CARTESIAN_POINT ( 'NONE',  ( -2.066987300000001415, 63.14382582708705627, 45.80000000109246372 ) ) ;
#18595=EDGE_CURVE ( 'NONE', #4896, #17611, #19143, .T. ) ;
#18602=CARTESIAN_POINT ( 'NONE',  ( 2.066987300000001415, 64.85617417291294373, 46.00000000109247367 ) ) ;
#18607=CARTESIAN_POINT ( 'NONE',  ( -0.8561741729129461742, 66.06698729999999387, 46.20000000109247651 ) ) ;
#18609=ORIENTED_EDGE ( 'NONE', *, *, #9935, .F. ) ;
#18611=CARTESIAN_POINT ( 'NONE',  ( -32.50000000000000000, 52.00000000000000711, 15.00000000000000000 ) ) ;
#18614=EDGE_CURVE ( 'NONE', #9379, #18899, #4273, .T. ) ;
#18625=EDGE_LOOP ( 'NONE', ( #4500, #8413, #8480, #611 ) ) ;
#18632=DIRECTION ( 'NONE',  ( -0.000000000000000000, -1.000000000000000000, -0.000000000000000000 ) ) ;
#18642=DIRECTION ( 'NONE',  ( -1.000000000000000000, 0.000000000000000000, -0.000000000000000000 ) ) ;
#18650=CARTESIAN_POINT ( 'NONE',  ( -1.035533905932738641, 66.50000000000000000, 49.85000000000000853 ) ) ;
#18660=ADVANCED_FACE ( 'NONE', ( #4339 ), #16193, .T. ) ;
#18662=CIRCLE ( 'NONE', #8023, 2.500000000000002220 ) ;
#18670=CARTESIAN_POINT ( 'NONE',  ( 2.500000000000001776, 65.03553390593273775, 45.75000000218494733 ) ) ;
#18674=CIRCLE ( 'NONE', #13324, 2.500000000000002220 ) ;
#18680=CARTESIAN_POINT ( 'NONE',  ( -0.8561741729129461742, 66.06698729999999387, 49.40000000109247225 ) ) ;
#18690=CARTESIAN_POINT ( 'NONE',  ( 1.767766952966369987, 65.76776695296638309, 48.89999999999999858 ) ) ;
#18702=CARTESIAN_POINT ( 'NONE',  ( -2.066987300000001859, 64.85617417291294373, 45.50000000109247367 ) ) ;
#18705=CARTESIAN_POINT ( 'NONE',  ( 2.500000000000001776, 64.00000000000000000, 45.70000000218494307 ) ) ;
#18714=ORIENTED_EDGE ( 'NONE', *, *, #12508, .F. ) ;
#18715=ORIENTED_EDGE ( 'NONE', *, *, #15601, .F. ) ;
#18724=ADVANCED_FACE ( 'NONE', ( #10296 ), #17869, .T. ) ;
#18731=FACE_OUTER_BOUND ( 'NONE', #18548, .T. ) ;
#18749=ORIENTED_EDGE ( 'NONE', *, *, #3755, .F. ) ;
#18750=CARTESIAN_POINT ( 'NONE',  ( -2.500000000000006661, 65.03553390593272354, 46.85000000218494165 ) ) ;
#18757=AXIS2_PLACEMENT_3D ( 'NONE', #14215, #782, #6767 ) ;
#18759=EDGE_CURVE ( 'NONE', #2559, #1624, #16591, .T. ) ;
#18763=CARTESIAN_POINT ( 'NONE',  ( 2.066987300000002303, 63.14382582708705627, 47.50000000109246656 ) ) ;
#18772=CARTESIAN_POINT ( 'NONE',  ( 1.767766952966370653, 62.23223304703363112, 48.69999999999999574 ) ) ;
#18773=CARTESIAN_POINT ( 'NONE',  ( -10.00000000000000000, -0.000000000000000000, 30.00000000000000000 ) ) ;
#18774=VECTOR ( 'NONE', #14143, 1000.000000000000000 ) ;
#18776=EDGE_CURVE ( 'NONE', #4687, #8924, #8965, .T. ) ;
#18780=AXIS2_PLACEMENT_3D ( 'NONE', #17949, #13619, #204 ) ;
#18782=CARTESIAN_POINT ( 'NONE',  ( -1.265664690411616068E-16, 66.06698730000000808, 46.15000000109247225 ) ) ;
#18784=ADVANCED_FACE ( 'NONE', ( #11773 ), #16289, .T. ) ;
#18788=CARTESIAN_POINT ( 'NONE',  ( -2.066987300000001415, 64.00000000000000000, 49.75000000109246656 ) ) ;
#18801=VERTEX_POINT ( 'NONE', #6501 ) ;
#18817=LINE ( 'NONE', #2530, #14419 ) ;
#18818=ORIENTED_EDGE ( 'NONE', *, *, #18941, .F. ) ;
#18821=CARTESIAN_POINT ( 'NONE',  ( 2.500000000000001776, 64.00000000000000000, 47.19999999999999574 ) ) ;
#18828=CARTESIAN_POINT ( 'NONE',  ( 2.500000000000002220, 62.96446609406726225, 47.25000000218494023 ) ) ;
#18844=LINE ( 'NONE', #11275, #17259 ) ;
#18858=FACE_OUTER_BOUND ( 'NONE', #14534, .T. ) ;
#18859=FACE_OUTER_BOUND ( 'NONE', #5769, .T. ) ;
#18866=CARTESIAN_POINT ( 'NONE',  ( 0.8561741729129460632, 66.06698729999999387, 49.30000000109246372 ) ) ;
#18868=CYLINDRICAL_SURFACE ( 'NONE', #5962, 2.499999999999998668 ) ;
#18869=CARTESIAN_POINT ( 'NONE',  ( 1.767766952966370653, 62.23223304703363112, 46.40000000218494591 ) ) ;
#18877=CARTESIAN_POINT ( 'NONE',  ( -2.066987300000001415, 63.14382582708705627, 45.00000000109246656 ) ) ;
#18878=CARTESIAN_POINT ( 'NONE',  ( -0.8561741729129461742, 66.06698730000000808, 49.60000000109247509 ) ) ;
#18889=CARTESIAN_POINT ( 'NONE',  ( -1.461580736456473906, 65.46158073645646880, 48.85000000109246798 ) ) ;
#18890=EDGE_CURVE ( 'NONE', #15274, #2308, #12462, .T. ) ;
#18899=VERTEX_POINT ( 'NONE', #4839 ) ;
#18910=CARTESIAN_POINT ( 'NONE',  ( -32.50000000000000000, 52.00000000000000711, -35.00000000000000000 ) ) ;
#18922=VERTEX_POINT ( 'NONE', #5030 ) ;
#18929=ORIENTED_EDGE ( 'NONE', *, *, #10203, .F. ) ;
#18933=CARTESIAN_POINT ( 'NONE',  ( 1.767766952966369987, 65.76776695296638309, 46.60000000218494165 ) ) ;
#18934=ORIENTED_EDGE ( 'NONE', *, *, #16240, .F. ) ;
#18941=EDGE_CURVE ( 'NONE', #3686, #9430, #6404, .T. ) ;
#18952=CARTESIAN_POINT ( 'NONE',  ( -2.066987300000001415, 64.00000000000000000, 49.55000000109247082 ) ) ;
#18961=CARTESIAN_POINT ( 'NONE',  ( -41.00000000000000000, 52.00000000000000711, 30.00000000000000000 ) ) ;
#18963=CARTESIAN_POINT ( 'NONE',  ( 3.796994071234847710E-16, 61.93301269999999903, 45.15000000109247225 ) ) ;
#18964=CARTESIAN_POINT ( 'NONE',  ( 1.461580736456473684, 65.46158073645646880, 48.65000000109247225 ) ) ;
#18973=CARTESIAN_POINT ( 'NONE',  ( -2.066987300000001415, 64.85617417291294373, 45.50000000109247367 ) ) ;
#18981=CARTESIAN_POINT ( 'NONE',  ( -1.461580736456473906, 65.46158073645646880, 47.25000000109246656 ) ) ;
#18987=DIRECTION ( 'NONE',  ( 0.000000000000000000, 1.000000000000000000, 0.000000000000000000 ) ) ;
#19006=( BOUNDED_CURVE ( )  B_SPLINE_CURVE ( 2, ( #18380, #13855, #618, #17004, #2095, #719, #7983, #16899, #6511 ),
 .UNSPECIFIED., .F., .F. ) 
 B_SPLINE_CURVE_WITH_KNOTS ( ( 3, 2, 2, 2, 3 ),
 ( 0.6428571428571427937, 0.6607142857142855874, 0.6785714285714284921, 0.6964285714285712858, 0.7142857142857141906 ),
 .UNSPECIFIED. ) 
 CURVE ( )  GEOMETRIC_REPRESENTATION_ITEM ( )  RATIONAL_B_SPLINE_CURVE ( ( 1.000000000000000444, 0.9238795325112862944, 1.000000000000000000, 0.9238795325112867385, 1.000000000000000000, 0.9238795325112867385, 1.000000000000000000, 0.9238795325112871826, 0.9999999999999995559 ) ) 
 REPRESENTATION_ITEM ( '' )  );
#19012=CARTESIAN_POINT ( 'NONE',  ( 2.500000000000001776, 64.00000000000000000, 49.99999999999999289 ) ) ;
#19015=LINE ( 'NONE', #13215, #6287 ) ;
#19020=ORIENTED_EDGE ( 'NONE', *, *, #12037, .F. ) ;
#19027=ORIENTED_EDGE ( 'NONE', *, *, #3062, .F. ) ;
#19029=( NAMED_UNIT ( * ) SI_UNIT ( $, .STERADIAN. ) SOLID_ANGLE_UNIT ( ) );
#19030=EDGE_LOOP ( 'NONE', ( #16395, #4723, #4715, #14001 ) ) ;
#19036=CARTESIAN_POINT ( 'NONE',  ( -2.500000000000001776, 64.00000000000000000, 48.50000000218494023 ) ) ;
#19045=CARTESIAN_POINT ( 'NONE',  ( -1.265664690411616068E-16, 66.06698730000000808, 46.95000000109246940 ) ) ;
#19054=DIRECTION ( 'NONE',  ( -0.000000000000000000, -0.000000000000000000, -1.000000000000000000 ) ) ;
#19056=CARTESIAN_POINT ( 'NONE',  ( 1.035533905932738197, 66.50000000000000000, 48.14999999999999858 ) ) ;
#19058=CIRCLE ( 'NONE', #3088, 2.999999999999999112 ) ;
#19070=AXIS2_PLACEMENT_3D ( 'NONE', #5771, #1663, #19302 ) ;
#19071=CARTESIAN_POINT ( 'NONE',  ( 0.8561741729129460632, 66.06698729999999387, 47.10000000109246798 ) ) ;
#19073=DIRECTION ( 'NONE',  ( 0.000000000000000000, 1.000000000000000000, -0.000000000000000000 ) ) ;
#19086=EDGE_LOOP ( 'NONE', ( #3369, #3438 ) ) ;
#19101=CARTESIAN_POINT ( 'NONE',  ( 24.00000000000000000, 47.00000000000000711, -67.72004514666936359 ) ) ;
#19102=ORIENTED_EDGE ( 'NONE', *, *, #15135, .T. ) ;
#19111=CARTESIAN_POINT ( 'NONE',  ( -3.999999999999996447, 47.00000000000000711, 30.00000000000000000 ) ) ;
#19113=CARTESIAN_POINT ( 'NONE',  ( -2.500000000000001776, 64.00000000000000000, 47.70000000218494307 ) ) ;
#19114=ORIENTED_EDGE ( 'NONE', *, *, #11287, .F. ) ;
#19123=AXIS2_PLACEMENT_3D ( 'NONE', #8309, #18987, #15762 ) ;
#19127=CARTESIAN_POINT ( 'NONE',  ( 2.499999999999996003, 65.03553390593275196, 48.85000000000000142 ) ) ;
#19134=DIRECTION ( 'NONE',  ( 0.000000000000000000, 0.000000000000000000, -1.000000000000000000 ) ) ;
#19135=CARTESIAN_POINT ( 'NONE',  ( -1.767766952966369765, 62.23223304703363112, 47.80000000218494449 ) ) ;
#19136=VECTOR ( 'NONE', #16584, 1000.000000000000000 ) ;
#19143=LINE ( 'NONE', #15727, #4587 ) ;
#19146=PRODUCT_DEFINITION ( 'UNKNOWN', '', #2978, #13346 ) ;
#19149=CARTESIAN_POINT ( 'NONE',  ( 2.066987300000002303, 63.14382582708705627, 45.10000000109246798 ) ) ;
#19151=AXIS2_PLACEMENT_3D ( 'NONE', #7675, #227, #12174 ) ;
#19154=FACE_BOUND ( 'NONE', #395, .T. ) ;
#19157=LINE ( 'NONE', #11489, #13457 ) ;
#19158=PLANE ( 'NONE',  #4990 ) ;
#19160=CARTESIAN_POINT ( 'NONE',  ( 1.035533905932739751, 61.50000000000000000, 46.24999999999998579 ) ) ;
#19161=CARTESIAN_POINT ( 'NONE',  ( 1.461580736456473684, 65.46158073645646880, 47.85000000109246798 ) ) ;
#19169=DIRECTION ( 'NONE',  ( -1.000000000000000000, -2.602085213965211135E-16, 0.000000000000000000 ) ) ;
#19171=CARTESIAN_POINT ( 'NONE',  ( 2.066987300000001415, 64.00000000000000000, 49.35000000109246798 ) ) ;
#19175=CARTESIAN_POINT ( 'NONE',  ( -1.461580736456473906, 65.46158073645646880, 49.65000000109246514 ) ) ;
#19177=EDGE_CURVE ( 'NONE', #4215, #18430, #8431, .T. ) ;
#19184=CARTESIAN_POINT ( 'NONE',  ( 1.035533905932739751, 61.50000000000000000, 44.75000000218494733 ) ) ;
#19188=EDGE_CURVE ( 'NONE', #4896, #5010, #7054, .T. ) ;
#19190=ORIENTED_EDGE ( 'NONE', *, *, #16240, .T. ) ;
#19191=ORIENTED_EDGE ( 'NONE', *, *, #12109, .F. ) ;
#19196=VERTEX_POINT ( 'NONE', #8344 ) ;
#19203=CARTESIAN_POINT ( 'NONE',  ( -32.50000000000000000, 52.00000000000000711, -35.00000000000000000 ) ) ;
#19211=ORIENTED_EDGE ( 'NONE', *, *, #3967, .T. ) ;
#19214=LINE ( 'NONE', #4316, #7091 ) ;
#19221=VERTEX_POINT ( 'NONE', #5692 ) ;
#19226=DIRECTION ( 'NONE',  ( -0.000000000000000000, -0.000000000000000000, -1.000000000000000000 ) ) ;
#19229=EDGE_CURVE ( 'NONE', #9140, #3001, #19214, .T. ) ;
#19233=DIRECTION ( 'NONE',  ( 0.000000000000000000, 0.000000000000000000, -1.000000000000000000 ) ) ;
#19235=CIRCLE ( 'NONE', #14228, 2.500000000000001776 ) ;
#19238=CARTESIAN_POINT ( 'NONE',  ( -41.00000000000000000, 0.000000000000000000, -50.00000000000000000 ) ) ;
#19244=CARTESIAN_POINT ( 'NONE',  ( -1.461580736456473906, 65.46158073645646880, 44.65000000109246514 ) ) ;
#19254=CARTESIAN_POINT ( 'NONE',  ( 4.592425496802577917E-16, 61.50000000000000000, 45.39999999999999858 ) ) ;
#19257=CARTESIAN_POINT ( 'NONE',  ( 1.767766952966370653, 62.23223304703363112, 47.09999999999999432 ) ) ;
#19258=CARTESIAN_POINT ( 'NONE',  ( 2.066987300000001415, 64.85617417291294373, 47.00000000109246656 ) ) ;
#19270=CARTESIAN_POINT ( 'NONE',  ( 2.066987300000002303, 63.14382582708705627, 46.10000000109246798 ) ) ;
#19272=AXIS2_PLACEMENT_3D ( 'NONE', #13636, #3451, #15507 ) ;
#19273=DIRECTION ( 'NONE',  ( 0.000000000000000000, 0.000000000000000000, -1.000000000000000000 ) ) ;
#19286=VECTOR ( 'NONE', #8183, 1000.000000000000000 ) ;
#19289=EDGE_LOOP ( 'NONE', ( #10381, #4093 ) ) ;
#19290=PRODUCT_DEFINITION_SHAPE ( 'NONE', 'NONE',  #19146 ) ;
#19297=VERTEX_POINT ( 'NONE', #14900 ) ;
#19299=CARTESIAN_POINT ( 'NONE',  ( 4.592425496802577917E-16, 61.50000000000000000, 46.99999999999999289 ) ) ;
#19302=DIRECTION ( 'NONE',  ( 6.123233995736588542E-17, -1.000000000000000000, 0.000000000000000000 ) ) ;
#19307=CARTESIAN_POINT ( 'NONE',  ( -14.99999999999999645, 52.00000000000000711, 23.99999999999997868 ) ) ;
#19314=DIRECTION ( 'NONE',  ( -2.602085213965211135E-16, 1.000000000000000000, -0.000000000000000000 ) ) ;
#19325=ORIENTED_EDGE ( 'NONE', *, *, #14452, .F. ) ;
#19327=ORIENTED_EDGE ( 'NONE', *, *, #17670, .F. ) ;
#19339=DIRECTION ( 'NONE',  ( 0.000000000000000000, 9.912705577010328508E-16, 1.000000000000000000 ) ) ;
#19343=CARTESIAN_POINT ( 'NONE',  ( -2.066987300000001415, 64.00000000000000000, 44.75000000109247367 ) ) ;
#19354=CARTESIAN_POINT ( 'NONE',  ( 2.066987300000001415, 64.85617417291294373, 46.20000000109248361 ) ) ;
#19355=EDGE_CURVE ( 'NONE', #3881, #4896, #17742, .T. ) ;
#19377=CARTESIAN_POINT ( 'NONE',  ( 3.999999999999998224, 67.00000000000000000, 34.99999999999999289 ) ) ;
#19389=CARTESIAN_POINT ( 'NONE',  ( 1.461580736456473906, 62.53841926354353120, 48.25000000109246656 ) ) ;
ENDSEC;
END-ISO-10303-21;
